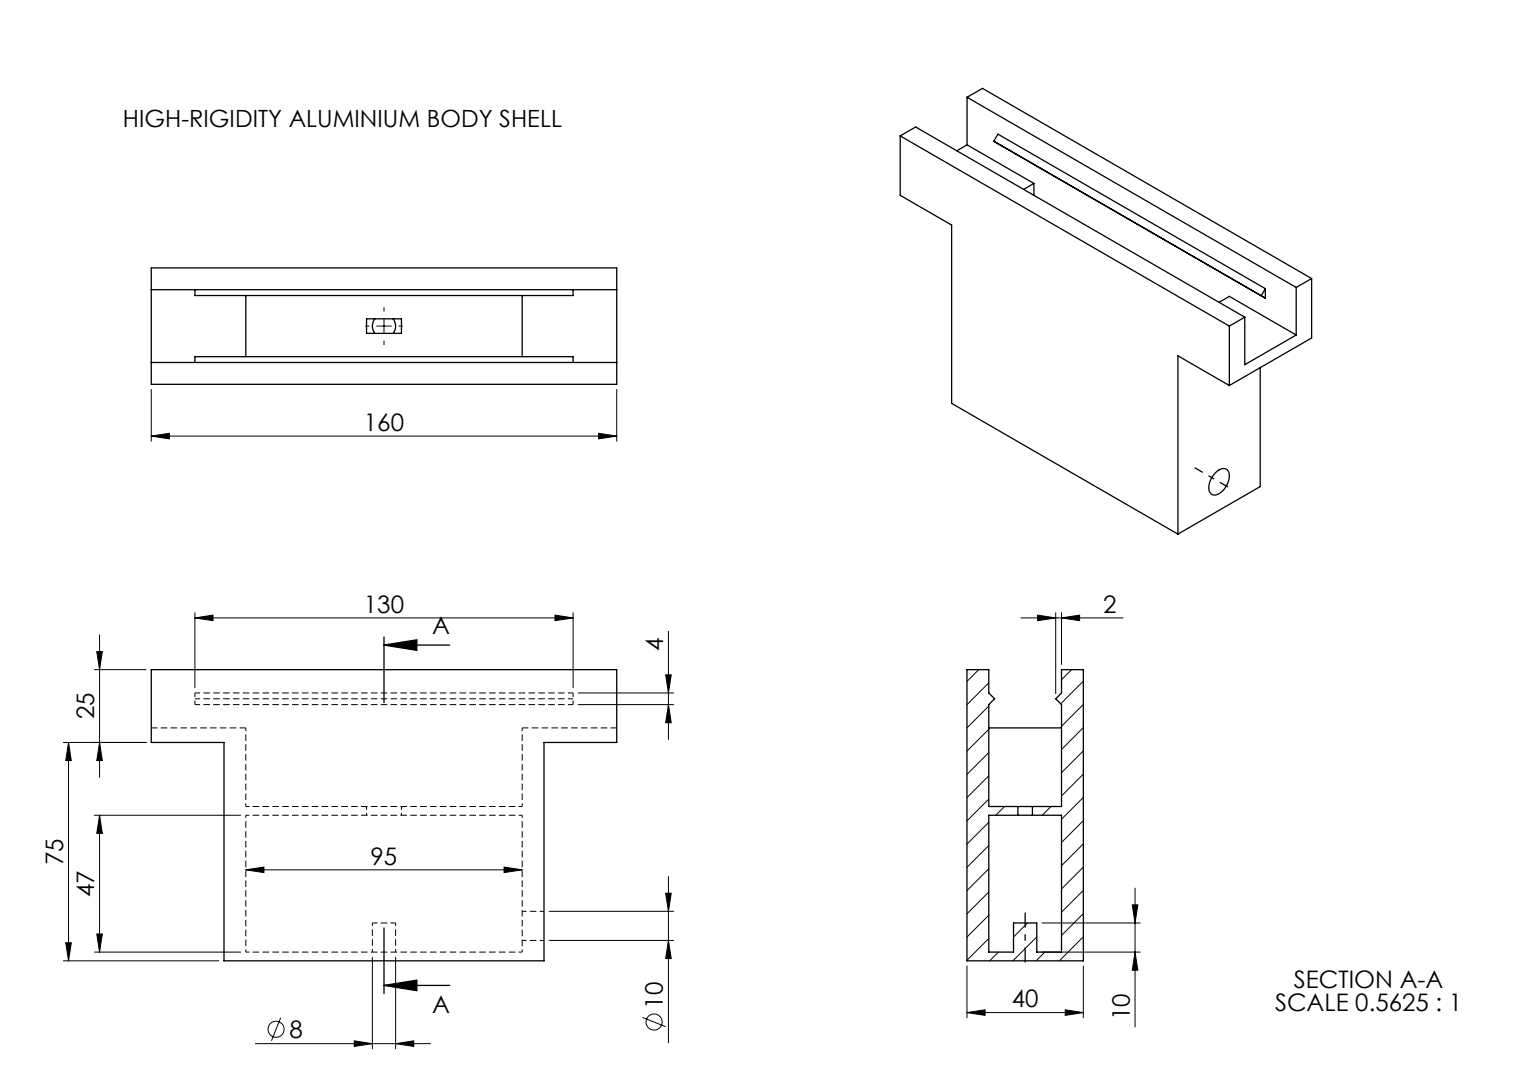
ISO-10303-21;
HEADER;
FILE_DESCRIPTION (('STEP AP214'),
    '1' );
FILE_NAME ('High-Rigidity Aluminium Body Shell.step',
    '2026-10-04T07:56:41',
    ( '' ),
    ( '' ),
    'SwSTEP 2.0',
    'SolidWorks 2026',
    '' );
FILE_SCHEMA (( 'AUTOMOTIVE_DESIGN' ));
ENDSEC;

DATA;
#5=LINE ( 'NONE', #7090, #369 ) ;
#14=LINE ( 'NONE', #7738, #5692 ) ;
#25=VECTOR ( 'NONE', #598, 1000.000000000000000 ) ;
#30=EDGE_LOOP ( 'NONE', ( #2065, #6214, #5997, #4915, #7865, #4258, #7605, #3266 ) ) ;
#39=CARTESIAN_POINT ( 'NONE',  ( -5.999999999999988454, -100.0010000000000048, -2.499999999999999112 ) ) ;
#47=FACE_OUTER_BOUND ( 'NONE', #854, .T. ) ;
#48=DIRECTION ( 'NONE',  ( -0.000000000000000000, 1.000000000000000000, 2.775557561562891351E-16 ) ) ;
#49=VECTOR ( 'NONE', #4022, 1000.000000000000000 ) ;
#50=AXIS2_PLACEMENT_3D ( 'NONE', #6623, #6543, #5905 ) ;
#52=EDGE_CURVE ( 'NONE', #1530, #5461, #2216, .T. ) ;
#56=ORIENTED_EDGE ( 'NONE', *, *, #5322, .F. ) ;
#58=LINE ( 'NONE', #6301, #4909 ) ;
#70=EDGE_CURVE ( 'NONE', #8240, #6658, #3048, .T. ) ;
#72=VERTEX_POINT ( 'NONE', #594 ) ;
#84=DIRECTION ( 'NONE',  ( 0.000000000000000000, -1.000000000000000000, -1.734723475976807094E-16 ) ) ;
#91=DIRECTION ( 'NONE',  ( 1.000000000000000000, -0.000000000000000000, -0.000000000000000000 ) ) ;
#94=ADVANCED_FACE ( 'NONE', ( #2381 ), #5021, .T. ) ;
#97=VERTEX_POINT ( 'NONE', #4421 ) ;
#98=AXIS2_PLACEMENT_3D ( 'NONE', #2797, #1653, #1018 ) ;
#107=LINE ( 'NONE', #2692, #5969 ) ;
#109=DIRECTION ( 'NONE',  ( -0.000000000000000000, 0.000000000000000000, -1.000000000000000000 ) ) ;
#113=EDGE_CURVE ( 'NONE', #4681, #4928, #8269, .T. ) ;
#114=ORIENTED_EDGE ( 'NONE', *, *, #1617, .T. ) ;
#119=ORIENTED_EDGE ( 'NONE', *, *, #70, .T. ) ;
#135=CARTESIAN_POINT ( 'NONE',  ( -65.00000000000000000, -7.999999999999992895, -12.50000000000000178 ) ) ;
#136=CARTESIAN_POINT ( 'NONE',  ( -65.00000000000000000, -12.00000000000000711, 12.49999999999999822 ) ) ;
#140=VERTEX_POINT ( 'NONE', #4384 ) ;
#145=CARTESIAN_POINT ( 'NONE',  ( -80.00000000000000000, -50.00000000000000711, -12.50000000000000888 ) ) ;
#146=CARTESIAN_POINT ( 'NONE',  ( 55.00000000000002132, -93.00000000000000000, 6.123233995736772199E-16 ) ) ;
#159=EDGE_LOOP ( 'NONE', ( #4079, #1702, #1986 ) ) ;
#160=FACE_OUTER_BOUND ( 'NONE', #6946, .T. ) ;
#167=EDGE_CURVE ( 'NONE', #2862, #1798, #3763, .T. ) ;
#170=CARTESIAN_POINT ( 'NONE',  ( 80.00000000000000000, 0.000000000000000000, 20.00000000000000000 ) ) ;
#176=CYLINDRICAL_SURFACE ( 'NONE', #6965, 5.000000000000004441 ) ;
#180=VECTOR ( 'NONE', #3060, 1000.000000000000000 ) ;
#184=VERTEX_POINT ( 'NONE', #4941 ) ;
#195=CARTESIAN_POINT ( 'NONE',  ( 80.00000000000000000, 0.000000000000000000, 20.00000000000000000 ) ) ;
#196=FILL_AREA_STYLE_COLOUR ( '', #1408 ) ;
#201=CARTESIAN_POINT ( 'NONE',  ( 80.00000000000000000, 0.000000000000000000, 20.00000000000000000 ) ) ;
#204=VERTEX_POINT ( 'NONE', #1706 ) ;
#211=DIRECTION ( 'NONE',  ( 9.251858538542971581E-17, -1.000000000000000000, 0.000000000000000000 ) ) ;
#216=CARTESIAN_POINT ( 'NONE',  ( -5.999999999999992895, -50.00000000000000000, -2.499999999999999112 ) ) ;
#217=DIRECTION ( 'NONE',  ( 0.000000000000000000, 0.7071067811865507924, -0.7071067811865441310 ) ) ;
#231=CARTESIAN_POINT ( 'NONE',  ( -80.00100000000001899, -83.00000000000002842, 0.000000000000000000 ) ) ;
#234=ORIENTED_EDGE ( 'NONE', *, *, #7378, .T. ) ;
#238=VERTEX_POINT ( 'NONE', #7087 ) ;
#239=DIRECTION ( 'NONE',  ( 0.000000000000000000, -0.000000000000000000, -1.000000000000000000 ) ) ;
#242=ORIENTED_EDGE ( 'NONE', *, *, #358, .F. ) ;
#251=FACE_OUTER_BOUND ( 'NONE', #7883, .T. ) ;
#255=AXIS2_PLACEMENT_3D ( 'NONE', #6696, #2244, #926 ) ;
#259=DIRECTION ( 'NONE',  ( 0.000000000000000000, 0.7071067811865442421, -0.7071067811865509034 ) ) ;
#262=ORIENTED_EDGE ( 'NONE', *, *, #5429, .F. ) ;
#267=VECTOR ( 'NONE', #2809, 1000.000000000000000 ) ;
#278=FILL_AREA_STYLE ('',( #196 ) ) ;
#281=ORIENTED_EDGE ( 'NONE', *, *, #3692, .F. ) ;
#282=DIRECTION ( 'NONE',  ( 0.000000000000000000, -2.775557561562891351E-16, 1.000000000000000000 ) ) ;
#285=ORIENTED_EDGE ( 'NONE', *, *, #8144, .T. ) ;
#303=FACE_OUTER_BOUND ( 'NONE', #1052, .T. ) ;
#308=ORIENTED_EDGE ( 'NONE', *, *, #7858, .F. ) ;
#312=CARTESIAN_POINT ( 'NONE',  ( -5.999999999999988454, -100.0010000000000048, 2.500000000000000888 ) ) ;
#320=ORIENTED_EDGE ( 'NONE', *, *, #4393, .F. ) ;
#321=CARTESIAN_POINT ( 'NONE',  ( 55.00000000000000000, -25.00000000000002132, 20.00000000000000000 ) ) ;
#339=CARTESIAN_POINT ( 'NONE',  ( 6.000000000000012434, -50.00000000000000000, 2.500000000000000888 ) ) ;
#343=ORIENTED_EDGE ( 'NONE', *, *, #113, .F. ) ;
#358=EDGE_CURVE ( 'NONE', #1800, #6097, #1314, .T. ) ;
#360=ORIENTED_EDGE ( 'NONE', *, *, #1284, .T. ) ;
#361=CYLINDRICAL_SURFACE ( 'NONE', #5299, 4.000000000000000000 ) ;
#369=VECTOR ( 'NONE', #5147, 1000.000000000000000 ) ;
#371=PRODUCT_CONTEXT ( 'NONE', #2292, 'mechanical' ) ;
#372=ORIENTED_EDGE ( 'NONE', *, *, #7078, .F. ) ;
#374=EDGE_CURVE ( 'NONE', #238, #5682, #7173, .T. ) ;
#375=ORIENTED_EDGE ( 'NONE', *, *, #3835, .T. ) ;
#379=LINE ( 'NONE', #7299, #1182 ) ;
#380=LINE ( 'NONE', #4853, #7186 ) ;
#382=CARTESIAN_POINT ( 'NONE',  ( -55.00000000000000000, -25.00000000000002132, 20.00000000000000000 ) ) ;
#383=EDGE_LOOP ( 'NONE', ( #4327, #3791, #8225, #2640 ) ) ;
#399=SURFACE_SIDE_STYLE ('',( #1115 ) ) ;
#401=ORIENTED_EDGE ( 'NONE', *, *, #6218, .F. ) ;
#403=ORIENTED_EDGE ( 'NONE', *, *, #1284, .F. ) ;
#415=ORIENTED_EDGE ( 'NONE', *, *, #5724, .T. ) ;
#416=CARTESIAN_POINT ( 'NONE',  ( 80.00000000000000000, 0.000000000000000000, 20.00000000000000000 ) ) ;
#421=DIRECTION ( 'NONE',  ( -1.261617073437677752E-16, 1.000000000000000000, 0.000000000000000000 ) ) ;
#434=DIRECTION ( 'NONE',  ( 0.000000000000000000, 0.000000000000000000, -1.000000000000000000 ) ) ;
#435=CIRCLE ( 'NONE', #50, 5.000000000000004441 ) ;
#438=EDGE_CURVE ( 'NONE', #4154, #6969, #4010, .T. ) ;
#442=EDGE_LOOP ( 'NONE', ( #7113, #2192, #7963, #2069 ) ) ;
#453=VECTOR ( 'NONE', #2497, 1000.000000000000000 ) ;
#455=EDGE_LOOP ( 'NONE', ( #5527, #7887, #7984, #6188 ) ) ;
#458=EDGE_LOOP ( 'NONE', ( #2051, #7413, #7304, #5700 ) ) ;
#467=ORIENTED_EDGE ( 'NONE', *, *, #5724, .F. ) ;
#483=LINE ( 'NONE', #2313, #180 ) ;
#493=ORIENTED_EDGE ( 'NONE', *, *, #657, .F. ) ;
#495=DIRECTION ( 'NONE',  ( -1.000000000000000000, -0.000000000000000000, -0.000000000000000000 ) ) ;
#508=EDGE_CURVE ( 'NONE', #4394, #4928, #3928, .T. ) ;
#525=DIRECTION ( 'NONE',  ( 1.261617073437677752E-16, -1.000000000000000000, -0.000000000000000000 ) ) ;
#550=DIRECTION ( 'NONE',  ( 0.000000000000000000, 0.000000000000000000, -1.000000000000000000 ) ) ;
#557=LINE ( 'NONE', #3220, #3294 ) ;
#578=LINE ( 'NONE', #2656, #3221 ) ;
#580=ORIENTED_EDGE ( 'NONE', *, *, #1489, .F. ) ;
#591=DIRECTION ( 'NONE',  ( -1.000000000000000000, -0.000000000000000000, -0.000000000000000000 ) ) ;
#594=CARTESIAN_POINT ( 'NONE',  ( -80.00000000000000000, 2.168404344971008868E-15, -12.50000000000000000 ) ) ;
#598=DIRECTION ( 'NONE',  ( -1.000000000000000000, -0.000000000000000000, -0.000000000000000000 ) ) ;
#604=VERTEX_POINT ( 'NONE', #826 ) ;
#613=CARTESIAN_POINT ( 'NONE',  ( -80.00000000000000000, -25.00000000000000000, 20.00000000000000000 ) ) ;
#619=CARTESIAN_POINT ( 'NONE',  ( -47.50000000000000711, -97.00000000000000000, 12.49999999999993960 ) ) ;
#628=CARTESIAN_POINT ( 'NONE',  ( 80.00000000000000000, 0.000000000000000000, 20.00000000000000000 ) ) ;
#636=LINE ( 'NONE', #5776, #2593 ) ;
#647=FACE_OUTER_BOUND ( 'NONE', #5300, .T. ) ;
#655=VECTOR ( 'NONE', #3803, 1000.000000000000000 ) ;
#657=EDGE_CURVE ( 'NONE', #72, #1757, #1333, .T. ) ;
#658=ORIENTED_EDGE ( 'NONE', *, *, #657, .T. ) ;
#659=FACE_BOUND ( 'NONE', #6052, .T. ) ;
#660=DIRECTION ( 'NONE',  ( -0.000000000000000000, -0.000000000000000000, -1.000000000000000000 ) ) ;
#669=EDGE_CURVE ( 'NONE', #1798, #1772, #3320, .T. ) ;
#681=CARTESIAN_POINT ( 'NONE',  ( -80.00000000000000000, 2.168404344971008868E-15, -12.50000000000000000 ) ) ;
#685=EDGE_LOOP ( 'NONE', ( #7292, #5717, #2988, #1427 ) ) ;
#687=CARTESIAN_POINT ( 'NONE',  ( 80.00000000000000000, -25.00000000000000000, 20.00000000000000000 ) ) ;
#688=CARTESIAN_POINT ( 'NONE',  ( -47.50000000000000711, -46.99999999999998579, -12.50000000000000888 ) ) ;
#702=CARTESIAN_POINT ( 'NONE',  ( -5.999999999999993783, -47.00000000000000000, -2.499999999999999112 ) ) ;
#716=VECTOR ( 'NONE', #6719, 1000.000000000000000 ) ;
#726=EDGE_CURVE ( 'NONE', #5175, #8255, #5334, .T. ) ;
#731=VERTEX_POINT ( 'NONE', #4655 ) ;
#747=LINE ( 'NONE', #4618, #7256 ) ;
#750=ORIENTED_EDGE ( 'NONE', *, *, #6561, .T. ) ;
#764=DIRECTION ( 'NONE',  ( -0.000000000000000000, -2.775557561562892337E-16, 1.000000000000000000 ) ) ;
#765=PLANE ( 'NONE',  #5548 ) ;
#769=ADVANCED_FACE ( 'NONE', ( #1502 ), #4069, .F. ) ;
#779=ADVANCED_FACE ( 'NONE', ( #5248 ), #6638, .F. ) ;
#792=CARTESIAN_POINT ( 'NONE',  ( 47.49999999999999289, -198.2344135219424857, 12.49999999999993960 ) ) ;
#794=ORIENTED_EDGE ( 'NONE', *, *, #5429, .T. ) ;
#806=EDGE_CURVE ( 'NONE', #6097, #3730, #5164, .T. ) ;
#807=LINE ( 'NONE', #39, #6725 ) ;
#821=DIRECTION ( 'NONE',  ( 1.000000000000000000, -0.000000000000000000, -0.000000000000000000 ) ) ;
#826=CARTESIAN_POINT ( 'NONE',  ( 80.00000000000000000, -25.00000000000000000, 20.00000000000000000 ) ) ;
#828=CARTESIAN_POINT ( 'NONE',  ( 80.00000000000000000, 2.168404344971008868E-15, -12.50000000000000000 ) ) ;
#843=EDGE_CURVE ( 'NONE', #7540, #3412, #107, .T. ) ;
#849=PLANE ( 'NONE',  #2666 ) ;
#850=CARTESIAN_POINT ( 'NONE',  ( 4.000000000000012434, -97.00000000000000000, 0.000000000000000000 ) ) ;
#854=EDGE_LOOP ( 'NONE', ( #4741, #415 ) ) ;
#861=CARTESIAN_POINT ( 'NONE',  ( 80.00000000000000000, 0.000000000000000000, 20.00000000000000000 ) ) ;
#864=VECTOR ( 'NONE', #7310, 1000.000000000000000 ) ;
#866=EDGE_CURVE ( 'NONE', #5004, #3412, #7048, .T. ) ;
#875=EDGE_LOOP ( 'NONE', ( #4314, #1494, #2609, #7246 ) ) ;
#888=FACE_OUTER_BOUND ( 'NONE', #2508, .T. ) ;
#894=LINE ( 'NONE', #136, #4759 ) ;
#898=ADVANCED_FACE ( 'NONE', ( #1362 ), #3345, .T. ) ;
#899=ORIENTED_EDGE ( 'NONE', *, *, #2957, .F. ) ;
#915=DIRECTION ( 'NONE',  ( 0.000000000000000000, 1.000000000000000000, 2.775557561562891351E-16 ) ) ;
#925=ORIENTED_EDGE ( 'NONE', *, *, #4635, .T. ) ;
#926=DIRECTION ( 'NONE',  ( -0.000000000000000000, 0.000000000000000000, -1.000000000000000000 ) ) ;
#932=VECTOR ( 'NONE', #2119, 1000.000000000000000 ) ;
#934=FACE_OUTER_BOUND ( 'NONE', #4950, .T. ) ;
#935=DIRECTION ( 'NONE',  ( 0.000000000000000000, -1.000000000000000000, 0.000000000000000000 ) ) ;
#948=DIRECTION ( 'NONE',  ( -1.000000000000000000, 0.000000000000000000, 0.000000000000000000 ) ) ;
#950=ADVANCED_FACE ( 'NONE', ( #47 ), #7770, .T. ) ;
#952=PLANE ( 'NONE',  #4975 ) ;
#954=ORIENTED_EDGE ( 'NONE', *, *, #8275, .F. ) ;
#956=ORIENTED_EDGE ( 'NONE', *, *, #4149, .T. ) ;
#961=ORIENTED_EDGE ( 'NONE', *, *, #806, .T. ) ;
#969=CARTESIAN_POINT ( 'NONE',  ( -5.999999999999988454, -100.0010000000000048, -2.499999999999999112 ) ) ;
#970=VERTEX_POINT ( 'NONE', #3218 ) ;
#974=EDGE_CURVE ( 'NONE', #4167, #3662, #5, .T. ) ;
#976=CARTESIAN_POINT ( 'NONE',  ( -80.00000000000000000, -47.00000000000000711, -12.50000000000000888 ) ) ;
#981=VERTEX_POINT ( 'NONE', #4551 ) ;
#982=LINE ( 'NONE', #2298, #7323 ) ;
#986=ORIENTED_EDGE ( 'NONE', *, *, #669, .T. ) ;
#991=EDGE_CURVE ( 'NONE', #2858, #7184, #5232, .T. ) ;
#994=VECTOR ( 'NONE', #495, 1000.000000000000000 ) ;
#1000=DIRECTION ( 'NONE',  ( -0.000000000000000000, 1.000000000000000000, 2.775557561562891351E-16 ) ) ;
#1012=VERTEX_POINT ( 'NONE', #135 ) ;
#1018=DIRECTION ( 'NONE',  ( 0.000000000000000000, -1.000000000000000000, -1.734723475976807094E-16 ) ) ;
#1023=EDGE_LOOP ( 'NONE', ( #7409, #4492, #6931, #3372 ) ) ;
#1024=CARTESIAN_POINT ( 'NONE',  ( 80.00000000000000000, 0.000000000000000000, -20.00000000000000000 ) ) ;
#1031=CARTESIAN_POINT ( 'NONE',  ( 47.49999999999999289, -46.99999999999998579, 12.49999999999998224 ) ) ;
#1032=ADVANCED_FACE ( 'NONE', ( #4469 ), #4594, .T. ) ;
#1034=( LENGTH_UNIT ( ) NAMED_UNIT ( * ) SI_UNIT ( .MILLI., .METRE. ) );
#1036=EDGE_LOOP ( 'NONE', ( #4830, #7266, #8107, #6146, #1939, #5954, #3636, #3435 ) ) ;
#1041=CARTESIAN_POINT ( 'NONE',  ( 1.223768561234547464E-14, -97.00000000000000000, 0.000000000000000000 ) ) ;
#1052=EDGE_LOOP ( 'NONE', ( #3029, #343, #320, #925 ) ) ;
#1062=EDGE_LOOP ( 'NONE', ( #5478, #3548, #403, #6706 ) ) ;
#1071=DIRECTION ( 'NONE',  ( -9.251858538542971581E-17, 1.000000000000000000, -0.000000000000000000 ) ) ;
#1076=ORIENTED_EDGE ( 'NONE', *, *, #1253, .F. ) ;
#1077=UNCERTAINTY_MEASURE_WITH_UNIT (LENGTH_MEASURE( 1.000000000000000082E-05 ), #5419, 'distance_accuracy_value', 'NONE');
#1090=ORIENTED_EDGE ( 'NONE', *, *, #3922, .T. ) ;
#1091=DIRECTION ( 'NONE',  ( -0.000000000000000000, -0.000000000000000000, -1.000000000000000000 ) ) ;
#1092=VERTEX_POINT ( 'NONE', #4012 ) ;
#1106=DIRECTION ( 'NONE',  ( -0.000000000000000000, -0.000000000000000000, -1.000000000000000000 ) ) ;
#1115=SURFACE_STYLE_FILL_AREA ( #8236 ) ;
#1118=ADVANCED_FACE ( 'NONE', ( #5950 ), #176, .F. ) ;
#1131=AXIS2_PLACEMENT_3D ( 'NONE', #7941, #259, #5193 ) ;
#1136=VERTEX_POINT ( 'NONE', #339 ) ;
#1158=PLANE ( 'NONE',  #2220 ) ;
#1162=VERTEX_POINT ( 'NONE', #216 ) ;
#1164=ADVANCED_FACE ( 'NONE', ( #4096, #7258 ), #4133, .F. ) ;
#1177=LINE ( 'NONE', #1816, #2009 ) ;
#1182=VECTOR ( 'NONE', #6075, 1000.000000000000000 ) ;
#1187=PLANE ( 'NONE',  #5298 ) ;
#1188=ORIENTED_EDGE ( 'NONE', *, *, #2399, .T. ) ;
#1189=LINE ( 'NONE', #3759, #453 ) ;
#1196=DIRECTION ( 'NONE',  ( 9.251858538542971581E-17, -1.000000000000000000, 0.000000000000000000 ) ) ;
#1197=VECTOR ( 'NONE', #5715, 1000.000000000000000 ) ;
#1202=VECTOR ( 'NONE', #84, 1000.000000000000000 ) ;
#1204=ADVANCED_FACE ( 'NONE', ( #1486 ), #849, .T. ) ;
#1206=VECTOR ( 'NONE', #2792, 1000.000000000000000 ) ;
#1232=DIRECTION ( 'NONE',  ( 0.000000000000000000, 0.000000000000000000, -1.000000000000000000 ) ) ;
#1245=CARTESIAN_POINT ( 'NONE',  ( -80.00000000000000000, -25.00000000000000000, 20.00000000000000000 ) ) ;
#1252=FACE_OUTER_BOUND ( 'NONE', #159, .T. ) ;
#1253=EDGE_CURVE ( 'NONE', #7447, #5257, #4677, .T. ) ;
#1260=ORIENTED_EDGE ( 'NONE', *, *, #358, .T. ) ;
#1275=DIRECTION ( 'NONE',  ( 0.000000000000000000, -1.000000000000000000, -1.734723475976807094E-16 ) ) ;
#1278=CARTESIAN_POINT ( 'NONE',  ( 55.00000000000000000, -25.00000000000002132, 20.00000000000000000 ) ) ;
#1279=CARTESIAN_POINT ( 'NONE',  ( -80.00000000000000000, -19.99999999999999645, -12.50000000000000355 ) ) ;
#1282=EDGE_LOOP ( 'NONE', ( #2510, #7406, #1561, #794 ) ) ;
#1284=EDGE_CURVE ( 'NONE', #6465, #5374, #5993, .T. ) ;
#1285=ORIENTED_EDGE ( 'NONE', *, *, #6456, .T. ) ;
#1300=LINE ( 'NONE', #619, #716 ) ;
#1314=LINE ( 'NONE', #3886, #1466 ) ;
#1318=LINE ( 'NONE', #3891, #25 ) ;
#1324=CARTESIAN_POINT ( 'NONE',  ( 80.00000000000000000, -25.00000000000000000, -20.00000000000000000 ) ) ;
#1331=VECTOR ( 'NONE', #6015, 1000.000000000000114 ) ;
#1333=LINE ( 'NONE', #4608, #1729 ) ;
#1336=LINE ( 'NONE', #1935, #7777 ) ;
#1341=VERTEX_POINT ( 'NONE', #6664 ) ;
#1342=LINE ( 'NONE', #702, #2282 ) ;
#1355=LINE ( 'NONE', #5898, #2705 ) ;
#1362=FACE_OUTER_BOUND ( 'NONE', #455, .T. ) ;
#1367=EDGE_LOOP ( 'NONE', ( #750, #4824, #5261, #5007 ) ) ;
#1370=CARTESIAN_POINT ( 'NONE',  ( -80.00000000000000000, 0.000000000000000000, 20.00000000000000000 ) ) ;
#1399=DIRECTION ( 'NONE',  ( -0.000000000000000000, -0.000000000000000000, -1.000000000000000000 ) ) ;
#1405=EDGE_CURVE ( 'NONE', #4928, #2966, #379, .T. ) ;
#1408=COLOUR_RGB ( '', 0.66274510, 0.83137255, 0.94901961) ;
#1412=DIRECTION ( 'NONE',  ( 1.000000000000000000, 9.251858538542971581E-17, 1.604941620322696727E-32 ) ) ;
#1422=CARTESIAN_POINT ( 'NONE',  ( -65.00000000000000000, -7.999999999999996447, 12.49999999999999822 ) ) ;
#1427=ORIENTED_EDGE ( 'NONE', *, *, #3922, .F. ) ;
#1431=ORIENTED_EDGE ( 'NONE', *, *, #1570, .T. ) ;
#1438=CARTESIAN_POINT ( 'NONE',  ( -80.00000000000000000, 2.168404344971008868E-15, -12.50000000000000000 ) ) ;
#1444=DIRECTION ( 'NONE',  ( 1.000000000000000000, 0.000000000000000000, 0.000000000000000000 ) ) ;
#1453=LINE ( 'NONE', #6594, #5169 ) ;
#1456=LINE ( 'NONE', #4028, #3228 ) ;
#1460=ADVANCED_FACE ( 'NONE', ( #934 ), #3467, .F. ) ;
#1466=VECTOR ( 'NONE', #1275, 1000.000000000000000 ) ;
#1467=ORIENTED_EDGE ( 'NONE', *, *, #3107, .T. ) ;
#1482=LINE ( 'NONE', #628, #7816 ) ;
#1486=FACE_OUTER_BOUND ( 'NONE', #1815, .T. ) ;
#1489=EDGE_CURVE ( 'NONE', #140, #2962, #8023, .T. ) ;
#1494=ORIENTED_EDGE ( 'NONE', *, *, #7223, .T. ) ;
#1502=FACE_OUTER_BOUND ( 'NONE', #6943, .T. ) ;
#1503=SURFACE_STYLE_FILL_AREA ( #278 ) ;
#1514=ADVANCED_FACE ( 'NONE', ( #4972 ), #1737, .F. ) ;
#1519=ORIENTED_EDGE ( 'NONE', *, *, #4696, .F. ) ;
#1521=DIRECTION ( 'NONE',  ( -1.000000000000000000, 0.000000000000000000, 0.000000000000000000 ) ) ;
#1522=FACE_OUTER_BOUND ( 'NONE', #685, .T. ) ;
#1529=AXIS2_PLACEMENT_3D ( 'NONE', #201, #8044, #239 ) ;
#1530=VERTEX_POINT ( 'NONE', #3713 ) ;
#1534=CIRCLE ( 'NONE', #5828, 4.000000000000000000 ) ;
#1550=ORIENTED_EDGE ( 'NONE', *, *, #4901, .F. ) ;
#1551=FACE_OUTER_BOUND ( 'NONE', #8281, .T. ) ;
#1554=VERTEX_POINT ( 'NONE', #6477 ) ;
#1561=ORIENTED_EDGE ( 'NONE', *, *, #167, .F. ) ;
#1570=EDGE_CURVE ( 'NONE', #1136, #981, #7746, .T. ) ;
#1571=UNCERTAINTY_MEASURE_WITH_UNIT (LENGTH_MEASURE( 1.000000000000000082E-05 ), #2347, 'distance_accuracy_value', 'NONE');
#1572=LINE ( 'NONE', #6791, #7584 ) ;
#1573=VERTEX_POINT ( 'NONE', #6434 ) ;
#1577=DIRECTION ( 'NONE',  ( -9.251858538542971581E-17, 1.000000000000000000, -0.000000000000000000 ) ) ;
#1582=EDGE_CURVE ( 'NONE', #7184, #3118, #1336, .T. ) ;
#1584=AXIS2_PLACEMENT_3D ( 'NONE', #3847, #5275, #1444 ) ;
#1588=( NAMED_UNIT ( * ) SI_UNIT ( $, .STERADIAN. ) SOLID_ANGLE_UNIT ( ) );
#1602=EDGE_LOOP ( 'NONE', ( #1188, #56, #2548, #7393 ) ) ;
#1609=ADVANCED_FACE ( 'NONE', ( #1252 ), #3947, .F. ) ;
#1610=VECTOR ( 'NONE', #6829, 1000.000000000000000 ) ;
#1617=EDGE_CURVE ( 'NONE', #3327, #7988, #5044, .T. ) ;
#1627=DIRECTION ( 'NONE',  ( -1.261617073437677752E-16, 1.000000000000000000, 0.000000000000000000 ) ) ;
#1633=DIRECTION ( 'NONE',  ( 0.000000000000000000, 0.7071067811865507924, -0.7071067811865441310 ) ) ;
#1635=DIRECTION ( 'NONE',  ( 0.000000000000000000, -1.000000000000000000, -1.734723475976807094E-16 ) ) ;
#1653=DIRECTION ( 'NONE',  ( 0.000000000000000000, -1.734723475976807094E-16, 1.000000000000000000 ) ) ;
#1663=VERTEX_POINT ( 'NONE', #3153 ) ;
#1668=ADVANCED_FACE ( 'NONE', ( #5709 ), #2518, .T. ) ;
#1679=DIRECTION ( 'NONE',  ( 1.000000000000000000, 0.000000000000000000, 0.000000000000000000 ) ) ;
#1687=ADVANCED_FACE ( 'NONE', ( #7025 ), #3824, .F. ) ;
#1692=FACE_OUTER_BOUND ( 'NONE', #30, .T. ) ;
#1702=ORIENTED_EDGE ( 'NONE', *, *, #2742, .F. ) ;
#1706=CARTESIAN_POINT ( 'NONE',  ( -65.00000000000000000, -12.00000000000000355, -12.50000000000000178 ) ) ;
#1729=VECTOR ( 'NONE', #7876, 1000.000000000000000 ) ;
#1737=PLANE ( 'NONE',  #3732 ) ;
#1742=FACE_OUTER_BOUND ( 'NONE', #1602, .T. ) ;
#1756=DIRECTION ( 'NONE',  ( 1.000000000000000000, 0.000000000000000000, 0.000000000000000000 ) ) ;
#1757=VERTEX_POINT ( 'NONE', #4071 ) ;
#1772=VERTEX_POINT ( 'NONE', #1422 ) ;
#1778=CARTESIAN_POINT ( 'NONE',  ( -54.99999999999999289, -100.0000000000000000, 20.00000000000000000 ) ) ;
#1783=CARTESIAN_POINT ( 'NONE',  ( 80.00000000000000000, -25.00000000000000000, 20.00000000000000000 ) ) ;
#1798=VERTEX_POINT ( 'NONE', #7959 ) ;
#1799=DIRECTION ( 'NONE',  ( -0.000000000000000000, 0.000000000000000000, 1.000000000000000000 ) ) ;
#1800=VERTEX_POINT ( 'NONE', #828 ) ;
#1802=DIRECTION ( 'NONE',  ( 1.000000000000000000, 1.261617073437677752E-16, 3.501690807976792361E-32 ) ) ;
#1815=EDGE_LOOP ( 'NONE', ( #2428, #308, #3461 ) ) ;
#1816=CARTESIAN_POINT ( 'NONE',  ( 65.00000000000000000, -9.999999999999994671, 10.50000000000000533 ) ) ;
#1826=CARTESIAN_POINT ( 'NONE',  ( -65.00000000000000000, -7.999999999999996447, 12.49999999999999822 ) ) ;
#1832=MANIFOLD_SOLID_BREP ( 'Cut-Extrude3', #1963 ) ;
#1844=ORIENTED_EDGE ( 'NONE', *, *, #4696, .T. ) ;
#1852=DIRECTION ( 'NONE',  ( -0.000000000000000000, 1.000000000000000000, 2.775557561562891351E-16 ) ) ;
#1863=AXIS2_PLACEMENT_3D ( 'NONE', #2604, #5880, #109 ) ;
#1878=VECTOR ( 'NONE', #1091, 1000.000000000000000 ) ;
#1880=EDGE_CURVE ( 'NONE', #5175, #2862, #2389, .T. ) ;
#1886=VECTOR ( 'NONE', #3859, 1000.000000000000000 ) ;
#1887=ORIENTED_EDGE ( 'NONE', *, *, #4926, .T. ) ;
#1888=CARTESIAN_POINT ( 'NONE',  ( 65.00000000000000000, -12.00000000000000355, -12.50000000000000178 ) ) ;
#1909=CARTESIAN_POINT ( 'NONE',  ( -80.00100000000001899, -93.00000000000004263, 6.123233995736772199E-16 ) ) ;
#1917=DIRECTION ( 'NONE',  ( 1.000000000000000000, 2.775557561562892337E-16, -0.000000000000000000 ) ) ;
#1935=CARTESIAN_POINT ( 'NONE',  ( 55.00000000000000000, -25.00000000000002132, 20.00000000000000000 ) ) ;
#1938=AXIS2_PLACEMENT_3D ( 'NONE', #2859, #915, #282 ) ;
#1939=ORIENTED_EDGE ( 'NONE', *, *, #7378, .F. ) ;
#1941=CARTESIAN_POINT ( 'NONE',  ( 65.00000000000000000, -7.999999999999992895, -12.50000000000000178 ) ) ;
#1962=DIRECTION ( 'NONE',  ( -1.000000000000000000, -1.261617073437677752E-16, -3.501690807976792361E-32 ) ) ;
#1963=CLOSED_SHELL ( 'NONE', ( #3411, #1032, #3271, #2345, #4211, #4487, #898, #6158, #3057, #5097, #7630, #779, #7010, #1164, #5712, #1460, #2041, #6132, #5943, #1687, #4380, #1514, #6128, #7098, #2710, #769, #5212, #5379, #94, #8306, #3727, #7921, #1668, #1609, #3609, #5284, #7576, #1204, #6288, #950, #1118 ) ) ;
#1968=CARTESIAN_POINT ( 'NONE',  ( 47.49999999999998579, -93.00000000000000000, 6.123233995736772199E-16 ) ) ;
#1970=DIRECTION ( 'NONE',  ( 0.000000000000000000, -0.000000000000000000, 1.000000000000000000 ) ) ;
#1983=DIRECTION ( 'NONE',  ( 0.000000000000000000, -1.000000000000000000, -1.734723475976807094E-16 ) ) ;
#1986=ORIENTED_EDGE ( 'NONE', *, *, #3601, .F. ) ;
#1995=CARTESIAN_POINT ( 'NONE',  ( 47.49999999999999289, -20.00000000000000355, 12.49999999999999112 ) ) ;
#2009=VECTOR ( 'NONE', #6944, 1000.000000000000000 ) ;
#2014=AXIS2_PLACEMENT_3D ( 'NONE', #8099, #2487, #4289 ) ;
#2041=ADVANCED_FACE ( 'NONE', ( #5501 ), #3649, .F. ) ;
#2051=ORIENTED_EDGE ( 'NONE', *, *, #6707, .F. ) ;
#2065=ORIENTED_EDGE ( 'NONE', *, *, #991, .T. ) ;
#2067=DIRECTION ( 'NONE',  ( -0.000000000000000000, 1.000000000000000000, 2.775557561562891351E-16 ) ) ;
#2069=ORIENTED_EDGE ( 'NONE', *, *, #2485, .T. ) ;
#2084=CARTESIAN_POINT ( 'NONE',  ( 55.00000000000002132, -82.99999999999998579, 0.000000000000000000 ) ) ;
#2095=CARTESIAN_POINT ( 'NONE',  ( 65.00000000000000000, -12.00000000000000355, -12.50000000000000178 ) ) ;
#2102=CARTESIAN_POINT ( 'NONE',  ( 65.00000000000000000, -7.999999999999996447, 12.49999999999999822 ) ) ;
#2119=DIRECTION ( 'NONE',  ( 1.000000000000000000, -0.000000000000000000, -0.000000000000000000 ) ) ;
#2124=DIRECTION ( 'NONE',  ( 1.000000000000000000, 9.251858538542971581E-17, 1.604941620322696727E-32 ) ) ;
#2133=ORIENTED_EDGE ( 'NONE', *, *, #5412, .F. ) ;
#2134=VECTOR ( 'NONE', #1852, 1000.000000000000000 ) ;
#2136=DIRECTION ( 'NONE',  ( -1.000000000000000000, -0.000000000000000000, -0.000000000000000000 ) ) ;
#2153=VERTEX_POINT ( 'NONE', #1968 ) ;
#2160=EDGE_LOOP ( 'NONE', ( #467, #6260, #1887, #3569 ) ) ;
#2162=PLANE ( 'NONE',  #7408 ) ;
#2171=EDGE_CURVE ( 'NONE', #5374, #2526, #3101, .T. ) ;
#2175=EDGE_LOOP ( 'NONE', ( #5491, #5086, #7142, #7162 ) ) ;
#2177=LINE ( 'NONE', #5411, #864 ) ;
#2192=ORIENTED_EDGE ( 'NONE', *, *, #70, .F. ) ;
#2201=LINE ( 'NONE', #3538, #932 ) ;
#2208=LINE ( 'NONE', #2839, #2619 ) ;
#2212=AXIS2_PLACEMENT_3D ( 'NONE', #321, #3995, #6684 ) ;
#2216=LINE ( 'NONE', #7351, #7943 ) ;
#2218=VECTOR ( 'NONE', #1071, 1000.000000000000000 ) ;
#2220=AXIS2_PLACEMENT_3D ( 'NONE', #6296, #1196, #7091 ) ;
#2222=AXIS2_PLACEMENT_3D ( 'NONE', #3044, #591, #550 ) ;
#2225=DIRECTION ( 'NONE',  ( -0.000000000000000000, -0.7071067811865507924, -0.7071067811865441310 ) ) ;
#2242=EDGE_CURVE ( 'NONE', #7184, #604, #2591, .T. ) ;
#2244=DIRECTION ( 'NONE',  ( 1.000000000000000000, 0.000000000000000000, -0.000000000000000000 ) ) ;
#2250=CARTESIAN_POINT ( 'NONE',  ( -80.00000000000000000, -47.00000000000000711, 12.49999999999999289 ) ) ;
#2256=DIRECTION ( 'NONE',  ( 1.000000000000000000, 0.000000000000000000, 0.000000000000000000 ) ) ;
#2263=DIRECTION ( 'NONE',  ( 0.000000000000000000, 0.000000000000000000, -1.000000000000000000 ) ) ;
#2266=CARTESIAN_POINT ( 'NONE',  ( 47.49999999999999289, -198.2344135219424857, -12.50000000000005151 ) ) ;
#2281=EDGE_CURVE ( 'NONE', #2962, #7308, #3774, .T. ) ;
#2282=VECTOR ( 'NONE', #6481, 1000.000000000000000 ) ;
#2283=ORIENTED_EDGE ( 'NONE', *, *, #7691, .T. ) ;
#2291=DIRECTION ( 'NONE',  ( 0.000000000000000000, 0.000000000000000000, 1.000000000000000000 ) ) ;
#2292=APPLICATION_CONTEXT ( 'automotive_design' ) ;
#2296=DIRECTION ( 'NONE',  ( 0.000000000000000000, 0.000000000000000000, -1.000000000000000000 ) ) ;
#2298=CARTESIAN_POINT ( 'NONE',  ( -80.00000000000000000, -2.168404344971008868E-15, 12.50000000000000000 ) ) ;
#2306=CARTESIAN_POINT ( 'NONE',  ( 6.000000000000007105, -50.00000000000000000, -2.499999999999999112 ) ) ;
#2311=DIRECTION ( 'NONE',  ( -1.000000000000000000, 0.000000000000000000, -0.000000000000000000 ) ) ;
#2313=CARTESIAN_POINT ( 'NONE',  ( -80.00000000000000000, -25.00000000000000000, -20.00000000000000000 ) ) ;
#2324=CARTESIAN_POINT ( 'NONE',  ( 6.000000000000006217, -47.00000000000000000, -2.499999999999999112 ) ) ;
#2343=AXIS2_PLACEMENT_3D ( 'NONE', #3856, #7147, #7610 ) ;
#2345=ADVANCED_FACE ( 'NONE', ( #5658, #7099 ), #6345, .T. ) ;
#2347=( LENGTH_UNIT ( ) NAMED_UNIT ( * ) SI_UNIT ( .MILLI., .METRE. ) );
#2352=UNCERTAINTY_MEASURE_WITH_UNIT (LENGTH_MEASURE( 1.000000000000000082E-05 ), #1034, 'distance_accuracy_value', 'NONE');
#2355=ORIENTED_EDGE ( 'NONE', *, *, #3890, .T. ) ;
#2367=ORIENTED_EDGE ( 'NONE', *, *, #3717, .T. ) ;
#2375=FACE_OUTER_BOUND ( 'NONE', #3074, .T. ) ;
#2376=ORIENTED_EDGE ( 'NONE', *, *, #7403, .F. ) ;
#2381=FACE_OUTER_BOUND ( 'NONE', #1036, .T. ) ;
#2389=LINE ( 'NONE', #4991, #7200 ) ;
#2391=DIRECTION ( 'NONE',  ( -1.261617073437677752E-16, 1.000000000000000000, 0.000000000000000000 ) ) ;
#2399=EDGE_CURVE ( 'NONE', #3118, #4154, #5737, .T. ) ;
#2404=CARTESIAN_POINT ( 'NONE',  ( 80.00000000000000000, -25.00000000000000000, 20.00000000000000000 ) ) ;
#2413=ORIENTED_EDGE ( 'NONE', *, *, #6523, .F. ) ;
#2419=CARTESIAN_POINT ( 'NONE',  ( -80.00000000000000000, -50.00000000000000711, 12.49999999999999289 ) ) ;
#2423=PLANE ( 'NONE',  #5437 ) ;
#2426=VECTOR ( 'NONE', #7312, 1000.000000000000000 ) ;
#2428=ORIENTED_EDGE ( 'NONE', *, *, #3717, .F. ) ;
#2429=EDGE_CURVE ( 'NONE', #1573, #7540, #58, .T. ) ;
#2432=FACE_OUTER_BOUND ( 'NONE', #3201, .T. ) ;
#2442=ORIENTED_EDGE ( 'NONE', *, *, #4590, .T. ) ;
#2443=FACE_OUTER_BOUND ( 'NONE', #1282, .T. ) ;
#2458=EDGE_CURVE ( 'NONE', #7988, #8240, #7187, .T. ) ;
#2464=DIRECTION ( 'NONE',  ( 0.000000000000000000, 0.000000000000000000, -1.000000000000000000 ) ) ;
#2485=EDGE_CURVE ( 'NONE', #7988, #2655, #5329, .T. ) ;
#2487=DIRECTION ( 'NONE',  ( 0.000000000000000000, 0.000000000000000000, -1.000000000000000000 ) ) ;
#2496=EDGE_LOOP ( 'NONE', ( #6830, #3490, #8007, #2721 ) ) ;
#2497=DIRECTION ( 'NONE',  ( -0.000000000000000000, 1.000000000000000000, 2.775557561562891351E-16 ) ) ;
#2508=EDGE_LOOP ( 'NONE', ( #7523, #6131, #8016, #5417 ) ) ;
#2510=ORIENTED_EDGE ( 'NONE', *, *, #4629, .T. ) ;
#2518=PLANE ( 'NONE',  #5073 ) ;
#2526=VERTEX_POINT ( 'NONE', #3477 ) ;
#2543=DIRECTION ( 'NONE',  ( 0.000000000000000000, -2.775557561562891351E-16, 1.000000000000000000 ) ) ;
#2548=ORIENTED_EDGE ( 'NONE', *, *, #2242, .F. ) ;
#2553=VECTOR ( 'NONE', #4545, 1000.000000000000000 ) ;
#2567=EDGE_LOOP ( 'NONE', ( #1431, #3511, #2951, #899 ) ) ;
#2568=CARTESIAN_POINT ( 'NONE',  ( -3.999999999999988898, -87.00000000000001421, 4.898587196589412829E-16 ) ) ;
#2570=ORIENTED_EDGE ( 'NONE', *, *, #6134, .T. ) ;
#2577=DIRECTION ( 'NONE',  ( 1.000000000000000000, -0.000000000000000000, -0.000000000000000000 ) ) ;
#2591=LINE ( 'NONE', #687, #3960 ) ;
#2593=VECTOR ( 'NONE', #1962, 1000.000000000000000 ) ;
#2601=DIRECTION ( 'NONE',  ( -9.251858538542971581E-17, 1.000000000000000000, 0.000000000000000000 ) ) ;
#2603=APPLICATION_CONTEXT ( 'automotive_design' ) ;
#2604=CARTESIAN_POINT ( 'NONE',  ( -65.00000000000000000, 0.000000000000000000, 0.000000000000000000 ) ) ;
#2608=VECTOR ( 'NONE', #3187, 1000.000000000000000 ) ;
#2609=ORIENTED_EDGE ( 'NONE', *, *, #843, .T. ) ;
#2619=VECTOR ( 'NONE', #935, 1000.000000000000000 ) ;
#2626=EDGE_CURVE ( 'NONE', #1554, #204, #7868, .T. ) ;
#2627=CARTESIAN_POINT ( 'NONE',  ( 65.00000000000000000, 0.000000000000000000, 0.000000000000000000 ) ) ;
#2640=ORIENTED_EDGE ( 'NONE', *, *, #113, .T. ) ;
#2643=LINE ( 'NONE', #1888, #6776 ) ;
#2654=EDGE_CURVE ( 'NONE', #5682, #970, #1453, .T. ) ;
#2655=VERTEX_POINT ( 'NONE', #3401 ) ;
#2656=CARTESIAN_POINT ( 'NONE',  ( -5.999999999999992895, -50.00000000000000000, -2.499999999999999112 ) ) ;
#2665=LINE ( 'NONE', #1438, #3761 ) ;
#2666=AXIS2_PLACEMENT_3D ( 'NONE', #3430, #2838, #6745 ) ;
#2680=EDGE_LOOP ( 'NONE', ( #281, #7421 ) ) ;
#2683=CIRCLE ( 'NONE', #5901, 4.000000000000000000 ) ;
#2692=CARTESIAN_POINT ( 'NONE',  ( -47.50000000000000711, -20.00000000000000355, 12.49999999999999112 ) ) ;
#2705=VECTOR ( 'NONE', #7719, 1000.000000000000000 ) ;
#2710=ADVANCED_FACE ( 'NONE', ( #5869 ), #6507, .F. ) ;
#2711=CARTESIAN_POINT ( 'NONE',  ( -54.99999999999999289, -100.0000000000000000, 20.00000000000000000 ) ) ;
#2712=CARTESIAN_POINT ( 'NONE',  ( -5.999999999999993783, -47.00000000000000000, -2.499999999999999112 ) ) ;
#2717=CARTESIAN_POINT ( 'NONE',  ( 1.097606853890779561E-14, -87.00000000000001421, 0.000000000000000000 ) ) ;
#2721=ORIENTED_EDGE ( 'NONE', *, *, #3407, .T. ) ;
#2742=EDGE_CURVE ( 'NONE', #1012, #2766, #2177, .T. ) ;
#2748=VECTOR ( 'NONE', #1802, 1000.000000000000000 ) ;
#2750=CARTESIAN_POINT ( 'NONE',  ( 1.223768561234547464E-14, -97.00000000000000000, 0.000000000000000000 ) ) ;
#2753=VECTOR ( 'NONE', #2296, 1000.000000000000000 ) ;
#2766=VERTEX_POINT ( 'NONE', #6800 ) ;
#2775=SURFACE_STYLE_USAGE ( .BOTH. , #6641 ) ;
#2790=ORIENTED_EDGE ( 'NONE', *, *, #7003, .F. ) ;
#2792=DIRECTION ( 'NONE',  ( -0.000000000000000000, -0.000000000000000000, -1.000000000000000000 ) ) ;
#2795=EDGE_CURVE ( 'NONE', #4167, #731, #1534, .T. ) ;
#2797=CARTESIAN_POINT ( 'NONE',  ( -80.00000000000000000, -2.168404344971008868E-15, 12.50000000000000000 ) ) ;
#2799=LINE ( 'NONE', #3431, #7705 ) ;
#2809=DIRECTION ( 'NONE',  ( -0.000000000000000000, 1.000000000000000000, 2.775557561562891351E-16 ) ) ;
#2821=EDGE_CURVE ( 'NONE', #1663, #5257, #8117, .T. ) ;
#2832=DIRECTION ( 'NONE',  ( 0.000000000000000000, 0.000000000000000000, 1.000000000000000000 ) ) ;
#2834=CARTESIAN_POINT ( 'NONE',  ( -80.00000000000000000, -25.00000000000000000, 20.00000000000000000 ) ) ;
#2838=DIRECTION ( 'NONE',  ( -1.000000000000000000, 0.000000000000000000, -0.000000000000000000 ) ) ;
#2839=CARTESIAN_POINT ( 'NONE',  ( -80.00000000000000000, 0.000000000000000000, -20.00000000000000000 ) ) ;
#2840=AXIS2_PLACEMENT_3D ( 'NONE', #8120, #5497, #1756 ) ;
#2858=VERTEX_POINT ( 'NONE', #8036 ) ;
#2859=CARTESIAN_POINT ( 'NONE',  ( -80.00000000000000000, -19.99999999999999645, -12.50000000000000355 ) ) ;
#2862=VERTEX_POINT ( 'NONE', #6880 ) ;
#2891=CARTESIAN_POINT ( 'NONE',  ( 1.097606853890779561E-14, -87.00000000000001421, 0.000000000000000000 ) ) ;
#2892=MECHANICAL_DESIGN_GEOMETRIC_PRESENTATION_REPRESENTATION('',(#8272),#3693);
#2900=CARTESIAN_POINT ( 'NONE',  ( -65.00000000000000000, -12.00000000000000355, -12.50000000000000178 ) ) ;
#2930=CARTESIAN_POINT ( 'NONE',  ( 55.00000000000002132, -99.99999999999998579, -20.00000000000000000 ) ) ;
#2932=VECTOR ( 'NONE', #2291, 1000.000000000000000 ) ;
#2938=PLANE ( 'NONE',  #6906 ) ;
#2948=SHAPE_DEFINITION_REPRESENTATION ( #3596, #7093 ) ;
#2951=ORIENTED_EDGE ( 'NONE', *, *, #52, .F. ) ;
#2954=VECTOR ( 'NONE', #6953, 1000.000000000000000 ) ;
#2957=EDGE_CURVE ( 'NONE', #1136, #1530, #4147, .T. ) ;
#2962=VERTEX_POINT ( 'NONE', #1031 ) ;
#2966=VERTEX_POINT ( 'NONE', #2930 ) ;
#2977=EDGE_LOOP ( 'NONE', ( #4835, #6883, #3718, #3019 ) ) ;
#2988=ORIENTED_EDGE ( 'NONE', *, *, #1570, .F. ) ;
#2989=LINE ( 'NONE', #3031, #7659 ) ;
#2990=ORIENTED_EDGE ( 'NONE', *, *, #7078, .T. ) ;
#3000=CARTESIAN_POINT ( 'NONE',  ( 55.00000000000000000, -25.00000000000002132, 20.00000000000000000 ) ) ;
#3008=DIRECTION ( 'NONE',  ( -1.000000000000000000, 0.000000000000000000, -0.000000000000000000 ) ) ;
#3014=ORIENTED_EDGE ( 'NONE', *, *, #6561, .F. ) ;
#3019=ORIENTED_EDGE ( 'NONE', *, *, #7634, .T. ) ;
#3029=ORIENTED_EDGE ( 'NONE', *, *, #508, .T. ) ;
#3031=CARTESIAN_POINT ( 'NONE',  ( -80.00000000000000000, -19.99999999999999645, -12.50000000000000355 ) ) ;
#3044=CARTESIAN_POINT ( 'NONE',  ( 47.49999999999998579, -88.00000000000000000, 0.000000000000000000 ) ) ;
#3048=LINE ( 'NONE', #2419, #655 ) ;
#3057=ADVANCED_FACE ( 'NONE', ( #7482 ), #2423, .F. ) ;
#3058=VECTOR ( 'NONE', #4488, 1000.000000000000000 ) ;
#3060=DIRECTION ( 'NONE',  ( 1.000000000000000000, -8.326672684688674053E-16, 0.000000000000000000 ) ) ;
#3074=EDGE_LOOP ( 'NONE', ( #114, #4062, #4119, #3349 ) ) ;
#3079=AXIS2_PLACEMENT_3D ( 'NONE', #969, #8017, #211 ) ;
#3086=VECTOR ( 'NONE', #7916, 1000.000000000000000 ) ;
#3101=LINE ( 'NONE', #6467, #7463 ) ;
#3107=EDGE_CURVE ( 'NONE', #72, #1573, #3767, .T. ) ;
#3118=VERTEX_POINT ( 'NONE', #4388 ) ;
#3125=LINE ( 'NONE', #5057, #1610 ) ;
#3127=DIRECTION ( 'NONE',  ( -1.000000000000000000, -8.326672684688674053E-16, 0.000000000000000000 ) ) ;
#3135=FACE_BOUND ( 'NONE', #4685, .T. ) ;
#3153=CARTESIAN_POINT ( 'NONE',  ( -5.999999999999992895, -50.00000000000000000, 2.500000000000001776 ) ) ;
#3158=ORIENTED_EDGE ( 'NONE', *, *, #3359, .T. ) ;
#3187=DIRECTION ( 'NONE',  ( 1.000000000000000000, 1.261617073437677752E-16, 0.000000000000000000 ) ) ;
#3194=DIRECTION ( 'NONE',  ( 8.326672684688674053E-16, 1.000000000000000000, -0.000000000000000000 ) ) ;
#3195=CARTESIAN_POINT ( 'NONE',  ( 6.000000000000011546, -100.0010000000000048, 2.500000000000000888 ) ) ;
#3201=EDGE_LOOP ( 'NONE', ( #3500, #119, #5362, #3158 ) ) ;
#3204=AXIS2_PLACEMENT_3D ( 'NONE', #681, #5775, #7814 ) ;
#3211=DIRECTION ( 'NONE',  ( -0.000000000000000000, 1.000000000000000000, -0.000000000000000000 ) ) ;
#3218=CARTESIAN_POINT ( 'NONE',  ( 80.00000000000000000, -2.168404344971008868E-15, 12.50000000000000000 ) ) ;
#3219=EDGE_CURVE ( 'NONE', #1573, #5004, #6417, .T. ) ;
#3220=CARTESIAN_POINT ( 'NONE',  ( 47.49999999999999289, -198.2344135219424857, 12.49999999999993960 ) ) ;
#3221=VECTOR ( 'NONE', #7751, 1000.000000000000000 ) ;
#3228=VECTOR ( 'NONE', #2225, 1000.000000000000114 ) ;
#3234=DIRECTION ( 'NONE',  ( -1.000000000000000000, -0.000000000000000000, -0.000000000000000000 ) ) ;
#3241=ORIENTED_EDGE ( 'NONE', *, *, #6456, .F. ) ;
#3242=FACE_OUTER_BOUND ( 'NONE', #3565, .T. ) ;
#3266=ORIENTED_EDGE ( 'NONE', *, *, #6508, .T. ) ;
#3269=EDGE_CURVE ( 'NONE', #2962, #5374, #6925, .T. ) ;
#3271=ADVANCED_FACE ( 'NONE', ( #3726, #3135 ), #1158, .T. ) ;
#3272=LINE ( 'NONE', #1370, #7722 ) ;
#3284=VECTOR ( 'NONE', #4315, 1000.000000000000000 ) ;
#3285=EDGE_LOOP ( 'NONE', ( #580, #956, #8162, #2790, #4169, #3956, #6303, #6820 ) ) ;
#3286=DIRECTION ( 'NONE',  ( 1.000000000000000000, -8.326672684688674053E-16, 0.000000000000000000 ) ) ;
#3294=VECTOR ( 'NONE', #48, 1000.000000000000000 ) ;
#3306=DIRECTION ( 'NONE',  ( -2.775557561562892337E-16, 1.000000000000000000, -0.000000000000000000 ) ) ;
#3307=CARTESIAN_POINT ( 'NONE',  ( 55.00000000000002132, -88.00000000000000000, 0.000000000000000000 ) ) ;
#3313=CARTESIAN_POINT ( 'NONE',  ( -47.50000000000000711, -49.99999999999998579, 12.49999999999993960 ) ) ;
#3315=LINE ( 'NONE', #5830, #2608 ) ;
#3317=DIRECTION ( 'NONE',  ( 0.000000000000000000, -0.7071067811865466846, -0.7071067811865484609 ) ) ;
#3320=LINE ( 'NONE', #2102, #6828 ) ;
#3325=EDGE_CURVE ( 'NONE', #4798, #6658, #557, .T. ) ;
#3327=VERTEX_POINT ( 'NONE', #3848 ) ;
#3345=PLANE ( 'NONE',  #3204 ) ;
#3349=ORIENTED_EDGE ( 'NONE', *, *, #4025, .T. ) ;
#3359=EDGE_CURVE ( 'NONE', #4798, #5382, #636, .T. ) ;
#3372=ORIENTED_EDGE ( 'NONE', *, *, #5640, .F. ) ;
#3376=ORIENTED_EDGE ( 'NONE', *, *, #1880, .T. ) ;
#3387=DIRECTION ( 'NONE',  ( -9.251858538542971581E-17, 1.000000000000000000, -0.000000000000000000 ) ) ;
#3401=CARTESIAN_POINT ( 'NONE',  ( 47.50000000000000000, -49.99999999999999289, -12.50000000000000888 ) ) ;
#3407=EDGE_CURVE ( 'NONE', #97, #2766, #1318, .T. ) ;
#3411=ADVANCED_FACE ( 'NONE', ( #8314 ), #5276, .F. ) ;
#3412=VERTEX_POINT ( 'NONE', #3468 ) ;
#3426=AXIS2_PLACEMENT_3D ( 'NONE', #382, #3510, #8027 ) ;
#3428=CIRCLE ( 'NONE', #2222, 5.000000000000004441 ) ;
#3430=CARTESIAN_POINT ( 'NONE',  ( -65.00000000000000000, 0.000000000000000000, 0.000000000000000000 ) ) ;
#3431=CARTESIAN_POINT ( 'NONE',  ( -65.00000000000000000, -12.00000000000000355, -12.50000000000000178 ) ) ;
#3435=ORIENTED_EDGE ( 'NONE', *, *, #3835, .F. ) ;
#3441=DIRECTION ( 'NONE',  ( -1.000000000000000000, 0.000000000000000000, 0.000000000000000000 ) ) ;
#3446=EDGE_LOOP ( 'NONE', ( #5213, #6347, #7281, #2570 ) ) ;
#3451=FACE_OUTER_BOUND ( 'NONE', #6987, .T. ) ;
#3461=ORIENTED_EDGE ( 'NONE', *, *, #4629, .F. ) ;
#3463=LINE ( 'NONE', #5520, #5915 ) ;
#3467=PLANE ( 'NONE',  #7371 ) ;
#3468=CARTESIAN_POINT ( 'NONE',  ( -47.50000000000000711, -20.00000000000000355, 12.49999999999999112 ) ) ;
#3472=EDGE_CURVE ( 'NONE', #6782, #3690, #6891, .T. ) ;
#3475=ORIENTED_EDGE ( 'NONE', *, *, #1880, .F. ) ;
#3477=CARTESIAN_POINT ( 'NONE',  ( 47.49999999999999289, -19.99999999999999645, -12.50000000000000000 ) ) ;
#3485=ORIENTED_EDGE ( 'NONE', *, *, #5515, .F. ) ;
#3490=ORIENTED_EDGE ( 'NONE', *, *, #2626, .F. ) ;
#3500=ORIENTED_EDGE ( 'NONE', *, *, #6196, .T. ) ;
#3505=DIRECTION ( 'NONE',  ( 1.000000000000000000, 0.000000000000000000, 0.000000000000000000 ) ) ;
#3506=PRODUCT_DEFINITION ( 'UNKNOWN', '', #7807, #6790 ) ;
#3510=DIRECTION ( 'NONE',  ( 1.000000000000000000, 9.251858538542972814E-17, -0.000000000000000000 ) ) ;
#3511=ORIENTED_EDGE ( 'NONE', *, *, #5697, .T. ) ;
#3538=CARTESIAN_POINT ( 'NONE',  ( -80.00000000000000000, -20.00000000000000355, 12.49999999999999645 ) ) ;
#3539=ORIENTED_EDGE ( 'NONE', *, *, #1582, .F. ) ;
#3548=ORIENTED_EDGE ( 'NONE', *, *, #3269, .T. ) ;
#3549=FACE_BOUND ( 'NONE', #4600, .T. ) ;
#3553=EDGE_LOOP ( 'NONE', ( #961, #8296, #2133, #4075, #4703, #7206, #401, #1260 ) ) ;
#3561=FILL_AREA_STYLE_COLOUR ( '', #8083 ) ;
#3565=EDGE_LOOP ( 'NONE', ( #5016, #360, #3777, #7028, #242, #1519, #1467, #7503 ) ) ;
#3566=FACE_OUTER_BOUND ( 'NONE', #3446, .T. ) ;
#3569=ORIENTED_EDGE ( 'NONE', *, *, #974, .F. ) ;
#3579=ORIENTED_EDGE ( 'NONE', *, *, #3325, .T. ) ;
#3587=CARTESIAN_POINT ( 'NONE',  ( 80.00000000000000000, -20.00000000000000355, 12.49999999999999645 ) ) ;
#3596=PRODUCT_DEFINITION_SHAPE ( 'NONE', 'NONE',  #3506 ) ;
#3601=EDGE_CURVE ( 'NONE', #204, #1012, #2799, .T. ) ;
#3603=VECTOR ( 'NONE', #2124, 1000.000000000000000 ) ;
#3604=( NAMED_UNIT ( * ) PLANE_ANGLE_UNIT ( ) SI_UNIT ( $, .RADIAN. ) );
#3606=ORIENTED_EDGE ( 'NONE', *, *, #167, .T. ) ;
#3609=ADVANCED_FACE ( 'NONE', ( #7857 ), #765, .F. ) ;
#3636=ORIENTED_EDGE ( 'NONE', *, *, #2399, .F. ) ;
#3648=ORIENTED_EDGE ( 'NONE', *, *, #2171, .F. ) ;
#3649=PLANE ( 'NONE',  #5699 ) ;
#3651=CARTESIAN_POINT ( 'NONE',  ( -47.50000000000000711, -198.2344135219424857, 12.49999999999993960 ) ) ;
#3662=VERTEX_POINT ( 'NONE', #850 ) ;
#3684=VECTOR ( 'NONE', #2067, 1000.000000000000000 ) ;
#3690=VERTEX_POINT ( 'NONE', #2084 ) ;
#3692=EDGE_CURVE ( 'NONE', #3690, #6782, #435, .T. ) ;
#3693=( GEOMETRIC_REPRESENTATION_CONTEXT ( 3 ) GLOBAL_UNCERTAINTY_ASSIGNED_CONTEXT ( ( #1077 ) ) GLOBAL_UNIT_ASSIGNED_CONTEXT ( ( #5419, #4610, #1588 ) ) REPRESENTATION_CONTEXT ( 'NONE', 'WORKASPACE' ) );
#3706=CARTESIAN_POINT ( 'NONE',  ( -5.999999999999993783, -47.00000000000000000, 2.500000000000000888 ) ) ;
#3708=ORIENTED_EDGE ( 'NONE', *, *, #5412, .T. ) ;
#3713=CARTESIAN_POINT ( 'NONE',  ( 6.000000000000012434, -50.00000000000000000, -2.499999999999999112 ) ) ;
#3717=EDGE_CURVE ( 'NONE', #8255, #184, #894, .T. ) ;
#3718=ORIENTED_EDGE ( 'NONE', *, *, #5762, .F. ) ;
#3726=FACE_OUTER_BOUND ( 'NONE', #442, .T. ) ;
#3727=ADVANCED_FACE ( 'NONE', ( #6034 ), #4639, .F. ) ;
#3730=VERTEX_POINT ( 'NONE', #3587 ) ;
#3732=AXIS2_PLACEMENT_3D ( 'NONE', #1778, #421, #7507 ) ;
#3751=VECTOR ( 'NONE', #7106, 1000.000000000000000 ) ;
#3753=VECTOR ( 'NONE', #2832, 1000.000000000000000 ) ;
#3759=CARTESIAN_POINT ( 'NONE',  ( -47.50000000000000711, -198.2344135219424857, -12.50000000000005151 ) ) ;
#3761=VECTOR ( 'NONE', #2577, 1000.000000000000000 ) ;
#3763=LINE ( 'NONE', #5569, #4827 ) ;
#3767=LINE ( 'NONE', #6964, #8264 ) ;
#3774=LINE ( 'NONE', #5033, #6781 ) ;
#3777=ORIENTED_EDGE ( 'NONE', *, *, #2171, .T. ) ;
#3791=ORIENTED_EDGE ( 'NONE', *, *, #3890, .F. ) ;
#3794=EDGE_CURVE ( 'NONE', #1757, #1341, #2208, .T. ) ;
#3799=CARTESIAN_POINT ( 'NONE',  ( -5.999999999999992895, -50.00000000000000000, -2.499999999999999112 ) ) ;
#3800=PLANE ( 'NONE',  #5832 ) ;
#3803=DIRECTION ( 'NONE',  ( 1.000000000000000000, 9.251858538542971581E-17, 1.604941620322696727E-32 ) ) ;
#3811=DIRECTION ( 'NONE',  ( 1.000000000000000000, 8.326672684688674053E-16, -0.000000000000000000 ) ) ;
#3824=PLANE ( 'NONE',  #4672 ) ;
#3829=ORIENTED_EDGE ( 'NONE', *, *, #4472, .T. ) ;
#3830=DIRECTION ( 'NONE',  ( 0.000000000000000000, -1.734723475976807094E-16, 1.000000000000000000 ) ) ;
#3831=CARTESIAN_POINT ( 'NONE',  ( 55.00000000000002132, -99.99999999999998579, 20.00000000000000000 ) ) ;
#3835=EDGE_CURVE ( 'NONE', #2966, #3118, #380, .T. ) ;
#3844=CARTESIAN_POINT ( 'NONE',  ( 80.00000000000000000, 0.000000000000000000, -20.00000000000000000 ) ) ;
#3847=CARTESIAN_POINT ( 'NONE',  ( 1.097606853890779561E-14, -87.00000000000001421, 0.000000000000000000 ) ) ;
#3848=CARTESIAN_POINT ( 'NONE',  ( -47.50000000000000711, -97.00000000000000000, -12.50000000000002309 ) ) ;
#3851=ORIENTED_EDGE ( 'NONE', *, *, #4049, .T. ) ;
#3856=CARTESIAN_POINT ( 'NONE',  ( 47.49999999999998579, -88.00000000000000000, 0.000000000000000000 ) ) ;
#3859=DIRECTION ( 'NONE',  ( -0.000000000000000000, -1.000000000000000000, -0.000000000000000000 ) ) ;
#3869=LINE ( 'NONE', #5845, #1197 ) ;
#3882=PLANE ( 'NONE',  #4036 ) ;
#3886=CARTESIAN_POINT ( 'NONE',  ( 80.00000000000000000, 2.168404344971008868E-15, -12.50000000000000000 ) ) ;
#3890=EDGE_CURVE ( 'NONE', #2858, #2966, #5049, .T. ) ;
#3891=CARTESIAN_POINT ( 'NONE',  ( 65.00000000000000000, -9.999999999999991118, -10.50000000000000888 ) ) ;
#3909=( GEOMETRIC_REPRESENTATION_CONTEXT ( 3 ) GLOBAL_UNCERTAINTY_ASSIGNED_CONTEXT ( ( #1571 ) ) GLOBAL_UNIT_ASSIGNED_CONTEXT ( ( #2347, #3604, #4913 ) ) REPRESENTATION_CONTEXT ( 'NONE', 'WORKASPACE' ) );
#3922=EDGE_CURVE ( 'NONE', #1663, #1136, #4450, .T. ) ;
#3928=LINE ( 'NONE', #5103, #4650 ) ;
#3947=PLANE ( 'NONE',  #1863 ) ;
#3954=FACE_OUTER_BOUND ( 'NONE', #6546, .T. ) ;
#3956=ORIENTED_EDGE ( 'NONE', *, *, #4829, .T. ) ;
#3960=VECTOR ( 'NONE', #7779, 1000.000000000000000 ) ;
#3985=CARTESIAN_POINT ( 'NONE',  ( 47.49999999999999289, -96.99999999999998579, -12.50000000000002309 ) ) ;
#3995=DIRECTION ( 'NONE',  ( -1.000000000000000000, -2.775557561562892337E-16, 0.000000000000000000 ) ) ;
#4010=LINE ( 'NONE', #3844, #8289 ) ;
#4012=CARTESIAN_POINT ( 'NONE',  ( 47.49999999999998579, -82.99999999999998579, 0.000000000000000000 ) ) ;
#4013=DIRECTION ( 'NONE',  ( -0.000000000000000000, 0.7071067811865442421, 0.7071067811865509034 ) ) ;
#4022=DIRECTION ( 'NONE',  ( 0.000000000000000000, 0.000000000000000000, 1.000000000000000000 ) ) ;
#4025=EDGE_CURVE ( 'NONE', #5382, #3327, #1300, .T. ) ;
#4028=CARTESIAN_POINT ( 'NONE',  ( 65.00000000000000000, -12.00000000000000355, -12.50000000000000178 ) ) ;
#4030=VECTOR ( 'NONE', #6370, 1000.000000000000000 ) ;
#4036=AXIS2_PLACEMENT_3D ( 'NONE', #2627, #4129, #4848 ) ;
#4049=EDGE_CURVE ( 'NONE', #4845, #1012, #4494, .T. ) ;
#4054=DIRECTION ( 'NONE',  ( 0.000000000000000000, 1.000000000000000000, 0.000000000000000000 ) ) ;
#4062=ORIENTED_EDGE ( 'NONE', *, *, #2458, .T. ) ;
#4069=PLANE ( 'NONE',  #5235 ) ;
#4071=CARTESIAN_POINT ( 'NONE',  ( -80.00000000000000000, 0.000000000000000000, -20.00000000000000000 ) ) ;
#4075=ORIENTED_EDGE ( 'NONE', *, *, #7555, .F. ) ;
#4076=CARTESIAN_POINT ( 'NONE',  ( 80.00000000000000000, -19.99999999999999645, -12.50000000000000355 ) ) ;
#4079=ORIENTED_EDGE ( 'NONE', *, *, #5897, .F. ) ;
#4096=FACE_BOUND ( 'NONE', #4448, .T. ) ;
#4100=DIRECTION ( 'NONE',  ( 9.251858538542972814E-17, -1.000000000000000000, 0.000000000000000000 ) ) ;
#4109=DIRECTION ( 'NONE',  ( 0.000000000000000000, 1.000000000000000000, 2.775557561562891351E-16 ) ) ;
#4115=PLANE ( 'NONE',  #2212 ) ;
#4119=ORIENTED_EDGE ( 'NONE', *, *, #6196, .F. ) ;
#4126=ORIENTED_EDGE ( 'NONE', *, *, #4926, .F. ) ;
#4128=PRODUCT ( 'High-Rigidity Aluminium Body Shell', 'High-Rigidity Aluminium Body Shell', '', ( #371 ) ) ;
#4129=DIRECTION ( 'NONE',  ( -1.000000000000000000, 0.000000000000000000, -0.000000000000000000 ) ) ;
#4133=PLANE ( 'NONE',  #98 ) ;
#4147=LINE ( 'NONE', #2306, #6510 ) ;
#4149=EDGE_CURVE ( 'NONE', #140, #3412, #4576, .T. ) ;
#4150=CARTESIAN_POINT ( 'NONE',  ( -65.00000000000000000, -12.00000000000000711, 12.49999999999999822 ) ) ;
#4154=VERTEX_POINT ( 'NONE', #5215 ) ;
#4167=VERTEX_POINT ( 'NONE', #7795 ) ;
#4169=ORIENTED_EDGE ( 'NONE', *, *, #2654, .T. ) ;
#4194=ORIENTED_EDGE ( 'NONE', *, *, #7858, .T. ) ;
#4206=EDGE_LOOP ( 'NONE', ( #3014, #372 ) ) ;
#4211=ADVANCED_FACE ( 'NONE', ( #7244, #3954 ), #6016, .F. ) ;
#4217=CARTESIAN_POINT ( 'NONE',  ( 47.49999999999999289, -49.99999999999998579, 12.49999999999993960 ) ) ;
#4219=ORIENTED_EDGE ( 'NONE', *, *, #2281, .T. ) ;
#4239=CARTESIAN_POINT ( 'NONE',  ( -80.00000000000000000, -2.168404344971008868E-15, 12.50000000000000000 ) ) ;
#4258=ORIENTED_EDGE ( 'NONE', *, *, #5762, .T. ) ;
#4259=LINE ( 'NONE', #8029, #7458 ) ;
#4287=AXIS2_PLACEMENT_3D ( 'NONE', #8294, #3830, #1983 ) ;
#4289=DIRECTION ( 'NONE',  ( -1.000000000000000000, 0.000000000000000000, -0.000000000000000000 ) ) ;
#4311=( NAMED_UNIT ( * ) SI_UNIT ( $, .STERADIAN. ) SOLID_ANGLE_UNIT ( ) );
#4314=ORIENTED_EDGE ( 'NONE', *, *, #4992, .F. ) ;
#4315=DIRECTION ( 'NONE',  ( -0.000000000000000000, -0.000000000000000000, -1.000000000000000000 ) ) ;
#4327=ORIENTED_EDGE ( 'NONE', *, *, #1405, .T. ) ;
#4337=DIRECTION ( 'NONE',  ( -0.000000000000000000, 0.000000000000000000, 1.000000000000000000 ) ) ;
#4343=DIRECTION ( 'NONE',  ( -1.000000000000000000, 0.000000000000000000, -0.000000000000000000 ) ) ;
#4354=AXIS2_PLACEMENT_3D ( 'NONE', #8108, #4902, #7474 ) ;
#4368=ORIENTED_EDGE ( 'NONE', *, *, #7634, .F. ) ;
#4369=CARTESIAN_POINT ( 'NONE',  ( 65.00000000000000000, -7.999999999999996447, 12.49999999999999822 ) ) ;
#4380=ADVANCED_FACE ( 'NONE', ( #303 ), #4513, .F. ) ;
#4384=CARTESIAN_POINT ( 'NONE',  ( -47.50000000000000711, -46.99999999999998579, 12.49999999999999112 ) ) ;
#4388=CARTESIAN_POINT ( 'NONE',  ( 55.00000000000000000, -25.00000000000002132, -20.00000000000000000 ) ) ;
#4393=EDGE_CURVE ( 'NONE', #7734, #4681, #1572, .T. ) ;
#4394=VERTEX_POINT ( 'NONE', #5361 ) ;
#4406=DIRECTION ( 'NONE',  ( -0.000000000000000000, -0.000000000000000000, -1.000000000000000000 ) ) ;
#4413=AXIS2_PLACEMENT_3D ( 'NONE', #4369, #7541, #8214 ) ;
#4421=CARTESIAN_POINT ( 'NONE',  ( 65.00000000000000000, -9.999999999999991118, -10.50000000000000888 ) ) ;
#4448=EDGE_LOOP ( 'NONE', ( #6609, #986, #4194, #6804 ) ) ;
#4449=CARTESIAN_POINT ( 'NONE',  ( -80.00000000000000000, -2.168404344971008868E-15, 12.50000000000000000 ) ) ;
#4450=LINE ( 'NONE', #6439, #8259 ) ;
#4469=FACE_OUTER_BOUND ( 'NONE', #2160, .T. ) ;
#4472=EDGE_CURVE ( 'NONE', #6658, #2655, #5486, .T. ) ;
#4487=ADVANCED_FACE ( 'NONE', ( #2375 ), #1187, .F. ) ;
#4488=DIRECTION ( 'NONE',  ( -9.251858538542971581E-17, 1.000000000000000000, -0.000000000000000000 ) ) ;
#4492=ORIENTED_EDGE ( 'NONE', *, *, #5753, .T. ) ;
#4494=LINE ( 'NONE', #1941, #994 ) ;
#4513=PLANE ( 'NONE',  #3426 ) ;
#4532=ORIENTED_EDGE ( 'NONE', *, *, #2742, .T. ) ;
#4533=CARTESIAN_POINT ( 'NONE',  ( 1.097606853890779561E-14, -87.00000000000001421, 0.000000000000000000 ) ) ;
#4545=DIRECTION ( 'NONE',  ( -1.000000000000000000, 0.000000000000000000, 0.000000000000000000 ) ) ;
#4551=CARTESIAN_POINT ( 'NONE',  ( 6.000000000000006217, -47.00000000000000000, 2.500000000000000888 ) ) ;
#4552=DIRECTION ( 'NONE',  ( 0.000000000000000000, 1.000000000000000000, 0.000000000000000000 ) ) ;
#4560=DIRECTION ( 'NONE',  ( -0.000000000000000000, 1.000000000000000000, 2.775557561562891351E-16 ) ) ;
#4562=DIRECTION ( 'NONE',  ( 0.000000000000000000, 1.000000000000000000, 0.000000000000000000 ) ) ;
#4576=LINE ( 'NONE', #6566, #3684 ) ;
#4590=EDGE_CURVE ( 'NONE', #1162, #1663, #5681, .T. ) ;
#4594=CYLINDRICAL_SURFACE ( 'NONE', #1584, 4.000000000000000000 ) ;
#4600=EDGE_LOOP ( 'NONE', ( #6668, #8043, #1076, #5565 ) ) ;
#4608=CARTESIAN_POINT ( 'NONE',  ( -80.00000000000000000, 0.000000000000000000, 20.00000000000000000 ) ) ;
#4610=( NAMED_UNIT ( * ) PLANE_ANGLE_UNIT ( ) SI_UNIT ( $, .RADIAN. ) );
#4618=CARTESIAN_POINT ( 'NONE',  ( -80.00000000000000000, -25.00000000000000000, 20.00000000000000000 ) ) ;
#4629=EDGE_CURVE ( 'NONE', #184, #1772, #8265, .T. ) ;
#4635=EDGE_CURVE ( 'NONE', #7734, #4394, #3125, .T. ) ;
#4639=PLANE ( 'NONE',  #1131 ) ;
#4650=VECTOR ( 'NONE', #6496, 1000.000000000000000 ) ;
#4655=CARTESIAN_POINT ( 'NONE',  ( -3.999999999999988898, -87.00000000000001421, 4.898587196589413815E-16 ) ) ;
#4672=AXIS2_PLACEMENT_3D ( 'NONE', #613, #3194, #6558 ) ;
#4677=LINE ( 'NONE', #7381, #2932 ) ;
#4681=VERTEX_POINT ( 'NONE', #2711 ) ;
#4685=EDGE_LOOP ( 'NONE', ( #1090, #6014, #8148, #2442 ) ) ;
#4689=VECTOR ( 'NONE', #1106, 1000.000000000000000 ) ;
#4692=CARTESIAN_POINT ( 'NONE',  ( -80.00000000000000000, -19.99999999999999645, -12.50000000000000355 ) ) ;
#4696=EDGE_CURVE ( 'NONE', #72, #1800, #2665, .T. ) ;
#4703=ORIENTED_EDGE ( 'NONE', *, *, #5322, .T. ) ;
#4704=PLANE ( 'NONE',  #1529 ) ;
#4705=DIRECTION ( 'NONE',  ( 1.000000000000000000, 0.000000000000000000, 0.000000000000000000 ) ) ;
#4715=DIRECTION ( 'NONE',  ( -0.000000000000000000, 0.000000000000000000, 1.000000000000000000 ) ) ;
#4722=EDGE_CURVE ( 'NONE', #5453, #238, #6410, .T. ) ;
#4733=CARTESIAN_POINT ( 'NONE',  ( -47.50000000000000711, -49.99999999999998579, 12.49999999999998224 ) ) ;
#4741=ORIENTED_EDGE ( 'NONE', *, *, #2795, .T. ) ;
#4759=VECTOR ( 'NONE', #217, 1000.000000000000114 ) ;
#4798=VERTEX_POINT ( 'NONE', #7083 ) ;
#4799=CARTESIAN_POINT ( 'NONE',  ( -54.99999999999999289, -100.0000000000000000, -20.00000000000000000 ) ) ;
#4805=DIRECTION ( 'NONE',  ( 1.000000000000000000, 9.251858538542971581E-17, 1.604941620322696727E-32 ) ) ;
#4815=ORIENTED_EDGE ( 'NONE', *, *, #6218, .T. ) ;
#4824=ORIENTED_EDGE ( 'NONE', *, *, #4901, .T. ) ;
#4827=VECTOR ( 'NONE', #4906, 1000.000000000000000 ) ;
#4829=EDGE_CURVE ( 'NONE', #970, #3730, #5896, .T. ) ;
#4830=ORIENTED_EDGE ( 'NONE', *, *, #1405, .F. ) ;
#4835=ORIENTED_EDGE ( 'NONE', *, *, #6258, .T. ) ;
#4845=VERTEX_POINT ( 'NONE', #7763 ) ;
#4846=PLANE ( 'NONE',  #255 ) ;
#4847=MECHANICAL_DESIGN_GEOMETRIC_PRESENTATION_REPRESENTATION('',(#6998),#3909);
#4848=DIRECTION ( 'NONE',  ( -0.000000000000000000, 0.000000000000000000, 1.000000000000000000 ) ) ;
#4853=CARTESIAN_POINT ( 'NONE',  ( 55.00000000000000000, -25.00000000000002132, -20.00000000000000000 ) ) ;
#4859=PLANE ( 'NONE',  #4354 ) ;
#4877=DIRECTION ( 'NONE',  ( -1.000000000000000000, 0.000000000000000000, 0.000000000000000000 ) ) ;
#4889=ORIENTED_EDGE ( 'NONE', *, *, #4722, .F. ) ;
#4890=LINE ( 'NONE', #2834, #1206 ) ;
#4901=EDGE_CURVE ( 'NONE', #2153, #6782, #7677, .T. ) ;
#4902=DIRECTION ( 'NONE',  ( 9.251858538542971581E-17, -1.000000000000000000, 0.000000000000000000 ) ) ;
#4906=DIRECTION ( 'NONE',  ( -0.000000000000000000, 0.7071067811865484609, 0.7071067811865465735 ) ) ;
#4909=VECTOR ( 'NONE', #5698, 1000.000000000000000 ) ;
#4913=( NAMED_UNIT ( * ) SI_UNIT ( $, .STERADIAN. ) SOLID_ANGLE_UNIT ( ) );
#4915=ORIENTED_EDGE ( 'NONE', *, *, #4722, .T. ) ;
#4926=EDGE_CURVE ( 'NONE', #7486, #3662, #6046, .T. ) ;
#4928=VERTEX_POINT ( 'NONE', #4799 ) ;
#4930=ORIENTED_EDGE ( 'NONE', *, *, #991, .F. ) ;
#4941=CARTESIAN_POINT ( 'NONE',  ( -65.00000000000000000, -9.999999999999994671, 10.50000000000000533 ) ) ;
#4950=EDGE_LOOP ( 'NONE', ( #7754, #4219, #7967, #3648 ) ) ;
#4972=FACE_OUTER_BOUND ( 'NONE', #383, .T. ) ;
#4975=AXIS2_PLACEMENT_3D ( 'NONE', #4692, #4109, #7954 ) ;
#4982=( GEOMETRIC_REPRESENTATION_CONTEXT ( 3 ) GLOBAL_UNCERTAINTY_ASSIGNED_CONTEXT ( ( #2352 ) ) GLOBAL_UNIT_ASSIGNED_CONTEXT ( ( #1034, #5538, #4311 ) ) REPRESENTATION_CONTEXT ( 'NONE', 'WORKASPACE' ) );
#4991=CARTESIAN_POINT ( 'NONE',  ( 65.00000000000000000, -12.00000000000000711, 12.49999999999999822 ) ) ;
#4992=EDGE_CURVE ( 'NONE', #6465, #140, #7422, .T. ) ;
#5004=VERTEX_POINT ( 'NONE', #7374 ) ;
#5007=ORIENTED_EDGE ( 'NONE', *, *, #8335, .F. ) ;
#5016=ORIENTED_EDGE ( 'NONE', *, *, #7223, .F. ) ;
#5021=PLANE ( 'NONE',  #7396 ) ;
#5031=VECTOR ( 'NONE', #3811, 1000.000000000000000 ) ;
#5033=CARTESIAN_POINT ( 'NONE',  ( 47.49999999999999289, -198.2344135219424857, 12.49999999999993960 ) ) ;
#5044=LINE ( 'NONE', #5749, #2134 ) ;
#5049=LINE ( 'NONE', #3831, #6775 ) ;
#5057=CARTESIAN_POINT ( 'NONE',  ( -55.00000000000000000, -25.00000000000002132, 20.00000000000000000 ) ) ;
#5058=ORIENTED_EDGE ( 'NONE', *, *, #806, .F. ) ;
#5071=DIRECTION ( 'NONE',  ( -1.000000000000000000, -1.261617073437677752E-16, 0.000000000000000000 ) ) ;
#5073=AXIS2_PLACEMENT_3D ( 'NONE', #5082, #5793, #7662 ) ;
#5075=DIRECTION ( 'NONE',  ( 0.000000000000000000, -1.000000000000000000, 0.000000000000000000 ) ) ;
#5082=CARTESIAN_POINT ( 'NONE',  ( 65.00000000000000000, 0.000000000000000000, 0.000000000000000000 ) ) ;
#5086=ORIENTED_EDGE ( 'NONE', *, *, #2429, .F. ) ;
#5089=ORIENTED_EDGE ( 'NONE', *, *, #5458, .F. ) ;
#5094=VECTOR ( 'NONE', #7623, 1000.000000000000000 ) ;
#5097=ADVANCED_FACE ( 'NONE', ( #888 ), #5311, .F. ) ;
#5103=CARTESIAN_POINT ( 'NONE',  ( -55.00000000000000000, -25.00000000000002132, -20.00000000000000000 ) ) ;
#5116=ORIENTED_EDGE ( 'NONE', *, *, #726, .T. ) ;
#5147=DIRECTION ( 'NONE',  ( 1.261617073437677752E-16, -1.000000000000000000, -0.000000000000000000 ) ) ;
#5154=DIRECTION ( 'NONE',  ( -1.261617073437677752E-16, 1.000000000000000000, 0.000000000000000000 ) ) ;
#5156=AXIS2_PLACEMENT_3D ( 'NONE', #861, #3441, #6674 ) ;
#5164=LINE ( 'NONE', #7743, #3751 ) ;
#5169=VECTOR ( 'NONE', #821, 1000.000000000000000 ) ;
#5171=ORIENTED_EDGE ( 'NONE', *, *, #3794, .T. ) ;
#5175=VERTEX_POINT ( 'NONE', #7293 ) ;
#5184=EDGE_CURVE ( 'NONE', #7308, #3730, #2201, .T. ) ;
#5189=DIRECTION ( 'NONE',  ( -0.000000000000000000, 1.000000000000000000, -0.000000000000000000 ) ) ;
#5192=DIRECTION ( 'NONE',  ( -1.261617073437677752E-16, 1.000000000000000000, 0.000000000000000000 ) ) ;
#5193=DIRECTION ( 'NONE',  ( 0.000000000000000000, 0.7071067811865507924, 0.7071067811865441310 ) ) ;
#5202=DIRECTION ( 'NONE',  ( 0.000000000000000000, 0.7071067811865483499, -0.7071067811865465735 ) ) ;
#5205=CARTESIAN_POINT ( 'NONE',  ( 65.00000000000000000, -12.00000000000000711, 12.49999999999999822 ) ) ;
#5212=ADVANCED_FACE ( 'NONE', ( #251 ), #4846, .F. ) ;
#5213=ORIENTED_EDGE ( 'NONE', *, *, #5522, .F. ) ;
#5215=CARTESIAN_POINT ( 'NONE',  ( 80.00000000000000000, -25.00000000000000000, -20.00000000000000000 ) ) ;
#5232=LINE ( 'NONE', #1278, #6297 ) ;
#5233=DIRECTION ( 'NONE',  ( 0.000000000000000000, 1.000000000000000000, 0.000000000000000000 ) ) ;
#5235=AXIS2_PLACEMENT_3D ( 'NONE', #195, #7152, #6556 ) ;
#5245=CARTESIAN_POINT ( 'NONE',  ( -47.50000000000000711, -49.99999999999998579, -12.50000000000001954 ) ) ;
#5248=FACE_OUTER_BOUND ( 'NONE', #2567, .T. ) ;
#5257=VERTEX_POINT ( 'NONE', #3706 ) ;
#5261=ORIENTED_EDGE ( 'NONE', *, *, #3472, .T. ) ;
#5275=DIRECTION ( 'NONE',  ( 1.261617073437677752E-16, -1.000000000000000000, -0.000000000000000000 ) ) ;
#5276=CYLINDRICAL_SURFACE ( 'NONE', #6626, 5.000000000000004441 ) ;
#5284=ADVANCED_FACE ( 'NONE', ( #2443 ), #6232, .F. ) ;
#5298=AXIS2_PLACEMENT_3D ( 'NONE', #7550, #6243, #4337 ) ;
#5299=AXIS2_PLACEMENT_3D ( 'NONE', #6886, #525, #1679 ) ;
#5300=EDGE_LOOP ( 'NONE', ( #4532, #5349, #2376, #3851 ) ) ;
#5311=PLANE ( 'NONE',  #3079 ) ;
#5318=CARTESIAN_POINT ( 'NONE',  ( -80.00100000000001899, -88.00000000000004263, 0.000000000000000000 ) ) ;
#5322=EDGE_CURVE ( 'NONE', #604, #4154, #6276, .T. ) ;
#5327=ORIENTED_EDGE ( 'NONE', *, *, #6707, .T. ) ;
#5329=LINE ( 'NONE', #145, #7054 ) ;
#5334=LINE ( 'NONE', #5205, #3086 ) ;
#5349=ORIENTED_EDGE ( 'NONE', *, *, #3407, .F. ) ;
#5358=DIRECTION ( 'NONE',  ( 0.000000000000000000, -0.7071067811865507924, 0.7071067811865441310 ) ) ;
#5361=CARTESIAN_POINT ( 'NONE',  ( -55.00000000000000000, -25.00000000000002132, -20.00000000000000000 ) ) ;
#5362=ORIENTED_EDGE ( 'NONE', *, *, #3325, .F. ) ;
#5374=VERTEX_POINT ( 'NONE', #7462 ) ;
#5379=ADVANCED_FACE ( 'NONE', ( #1692 ), #6819, .F. ) ;
#5382=VERTEX_POINT ( 'NONE', #7578 ) ;
#5393=ORIENTED_EDGE ( 'NONE', *, *, #5184, .T. ) ;
#5399=CARTESIAN_POINT ( 'NONE',  ( 47.49999999999999289, -198.2344135219424857, 12.49999999999993960 ) ) ;
#5411=CARTESIAN_POINT ( 'NONE',  ( -65.00000000000000000, -7.999999999999992895, -12.50000000000000178 ) ) ;
#5412=EDGE_CURVE ( 'NONE', #5453, #970, #5593, .T. ) ;
#5414=LINE ( 'NONE', #231, #2426 ) ;
#5417=ORIENTED_EDGE ( 'NONE', *, *, #4590, .F. ) ;
#5418=AXIS2_PLACEMENT_3D ( 'NONE', #3307, #7221, #4552 ) ;
#5419=( LENGTH_UNIT ( ) NAMED_UNIT ( * ) SI_UNIT ( .MILLI., .METRE. ) );
#5425=ORIENTED_EDGE ( 'NONE', *, *, #3107, .F. ) ;
#5429=EDGE_CURVE ( 'NONE', #2862, #184, #1177, .T. ) ;
#5433=VECTOR ( 'NONE', #1000, 1000.000000000000000 ) ;
#5437=AXIS2_PLACEMENT_3D ( 'NONE', #6839, #434, #3008 ) ;
#5438=DIRECTION ( 'NONE',  ( 1.000000000000000000, 0.000000000000000000, 0.000000000000000000 ) ) ;
#5453=VERTEX_POINT ( 'NONE', #416 ) ;
#5458=EDGE_CURVE ( 'NONE', #2526, #6097, #2989, .T. ) ;
#5461=VERTEX_POINT ( 'NONE', #2324 ) ;
#5478=ORIENTED_EDGE ( 'NONE', *, *, #1489, .T. ) ;
#5486=LINE ( 'NONE', #4217, #2753 ) ;
#5491=ORIENTED_EDGE ( 'NONE', *, *, #843, .F. ) ;
#5497=DIRECTION ( 'NONE',  ( 0.000000000000000000, 0.000000000000000000, 1.000000000000000000 ) ) ;
#5500=VECTOR ( 'NONE', #4406, 1000.000000000000000 ) ;
#5501=FACE_OUTER_BOUND ( 'NONE', #875, .T. ) ;
#5505=CARTESIAN_POINT ( 'NONE',  ( 80.00000000000000000, 0.000000000000000000, 20.00000000000000000 ) ) ;
#5515=EDGE_CURVE ( 'NONE', #7308, #2526, #6900, .T. ) ;
#5520=CARTESIAN_POINT ( 'NONE',  ( 65.00000000000000000, -12.00000000000000711, 12.49999999999999822 ) ) ;
#5522=EDGE_CURVE ( 'NONE', #731, #7486, #5556, .T. ) ;
#5527=ORIENTED_EDGE ( 'NONE', *, *, #2485, .F. ) ;
#5528=FACE_OUTER_BOUND ( 'NONE', #1062, .T. ) ;
#5538=( NAMED_UNIT ( * ) PLANE_ANGLE_UNIT ( ) SI_UNIT ( $, .RADIAN. ) );
#5548=AXIS2_PLACEMENT_3D ( 'NONE', #7902, #4013, #5358 ) ;
#5556=LINE ( 'NONE', #2568, #5626 ) ;
#5559=AXIS2_PLACEMENT_3D ( 'NONE', #1041, #2391, #4877 ) ;
#5565=ORIENTED_EDGE ( 'NONE', *, *, #5753, .F. ) ;
#5569=CARTESIAN_POINT ( 'NONE',  ( 65.00000000000000000, -7.999999999999996447, 12.49999999999999822 ) ) ;
#5593=LINE ( 'NONE', #5634, #1878 ) ;
#5626=VECTOR ( 'NONE', #6525, 1000.000000000000000 ) ;
#5634=CARTESIAN_POINT ( 'NONE',  ( 80.00000000000000000, 0.000000000000000000, 20.00000000000000000 ) ) ;
#5640=EDGE_CURVE ( 'NONE', #1530, #1162, #578, .T. ) ;
#5656=SURFACE_STYLE_USAGE ( .BOTH. , #399 ) ;
#5658=FACE_BOUND ( 'NONE', #6568, .T. ) ;
#5659=ORIENTED_EDGE ( 'NONE', *, *, #7003, .T. ) ;
#5671=CARTESIAN_POINT ( 'NONE',  ( 47.49999999999999289, -20.00000000000000355, 12.49999999999999112 ) ) ;
#5681=LINE ( 'NONE', #3799, #4030 ) ;
#5682=VERTEX_POINT ( 'NONE', #4449 ) ;
#5692=VECTOR ( 'NONE', #1970, 1000.000000000000000 ) ;
#5697=EDGE_CURVE ( 'NONE', #981, #5461, #3869, .T. ) ;
#5698=DIRECTION ( 'NONE',  ( 1.000000000000000000, -0.000000000000000000, -0.000000000000000000 ) ) ;
#5699=AXIS2_PLACEMENT_3D ( 'NONE', #6884, #2311, #1799 ) ;
#5700=ORIENTED_EDGE ( 'NONE', *, *, #3359, .F. ) ;
#5709=FACE_OUTER_BOUND ( 'NONE', #7229, .T. ) ;
#5712=ADVANCED_FACE ( 'NONE', ( #659, #3242 ), #5798, .T. ) ;
#5715=DIRECTION ( 'NONE',  ( -0.000000000000000000, -0.000000000000000000, -1.000000000000000000 ) ) ;
#5717=ORIENTED_EDGE ( 'NONE', *, *, #6924, .T. ) ;
#5724=EDGE_CURVE ( 'NONE', #731, #4167, #2683, .T. ) ;
#5737=LINE ( 'NONE', #1324, #5031 ) ;
#5749=CARTESIAN_POINT ( 'NONE',  ( -47.50000000000000711, -198.2344135219424857, -12.50000000000005151 ) ) ;
#5753=EDGE_CURVE ( 'NONE', #5461, #7447, #1342, .T. ) ;
#5762=EDGE_CURVE ( 'NONE', #6651, #7734, #747, .T. ) ;
#5769=FACE_OUTER_BOUND ( 'NONE', #6695, .T. ) ;
#5775=DIRECTION ( 'NONE',  ( 0.000000000000000000, -1.734723475976807094E-16, 1.000000000000000000 ) ) ;
#5776=CARTESIAN_POINT ( 'NONE',  ( -47.50000000000002132, -97.00000000000000000, 12.49999999999996803 ) ) ;
#5788=PLANE ( 'NONE',  #8078 ) ;
#5791=CARTESIAN_POINT ( 'NONE',  ( 6.000000000000011546, -100.0010000000000048, -2.499999999999999112 ) ) ;
#5793=DIRECTION ( 'NONE',  ( 1.000000000000000000, 0.000000000000000000, -0.000000000000000000 ) ) ;
#5798=PLANE ( 'NONE',  #4287 ) ;
#5825=CARTESIAN_POINT ( 'NONE',  ( -54.99999999999999289, -97.00000000000000000, 20.00000000000000000 ) ) ;
#5828=AXIS2_PLACEMENT_3D ( 'NONE', #2891, #1627, #948 ) ;
#5830=CARTESIAN_POINT ( 'NONE',  ( -54.99999999999999289, -100.0000000000000000, 20.00000000000000000 ) ) ;
#5832=AXIS2_PLACEMENT_3D ( 'NONE', #1783, #7636, #3127 ) ;
#5845=CARTESIAN_POINT ( 'NONE',  ( 6.000000000000006217, -47.00000000000000000, -2.499999999999999112 ) ) ;
#5856=LINE ( 'NONE', #6536, #2553 ) ;
#5862=CARTESIAN_POINT ( 'NONE',  ( -80.00000000000000000, -20.00000000000000355, 12.49999999999999645 ) ) ;
#5869=FACE_OUTER_BOUND ( 'NONE', #3553, .T. ) ;
#5880=DIRECTION ( 'NONE',  ( 1.000000000000000000, 0.000000000000000000, -0.000000000000000000 ) ) ;
#5896=LINE ( 'NONE', #7717, #1202 ) ;
#5897=EDGE_CURVE ( 'NONE', #2766, #204, #8004, .T. ) ;
#5898=CARTESIAN_POINT ( 'NONE',  ( 65.00000000000000000, -7.999999999999992895, -12.50000000000000178 ) ) ;
#5901=AXIS2_PLACEMENT_3D ( 'NONE', #4533, #7114, #7029 ) ;
#5905=DIRECTION ( 'NONE',  ( 0.000000000000000000, 1.000000000000000000, 0.000000000000000000 ) ) ;
#5915=VECTOR ( 'NONE', #6618, 1000.000000000000000 ) ;
#5943=ADVANCED_FACE ( 'NONE', ( #160 ), #4704, .F. ) ;
#5950=FACE_OUTER_BOUND ( 'NONE', #7464, .T. ) ;
#5954=ORIENTED_EDGE ( 'NONE', *, *, #438, .F. ) ;
#5957=ORIENTED_EDGE ( 'NONE', *, *, #4049, .F. ) ;
#5969=VECTOR ( 'NONE', #764, 1000.000000000000000 ) ;
#5983=AXIS2_PLACEMENT_3D ( 'NONE', #5825, #5154, #5071 ) ;
#5993=LINE ( 'NONE', #976, #3603 ) ;
#5997=ORIENTED_EDGE ( 'NONE', *, *, #7555, .T. ) ;
#6006=LINE ( 'NONE', #2266, #267 ) ;
#6014=ORIENTED_EDGE ( 'NONE', *, *, #2957, .T. ) ;
#6015=DIRECTION ( 'NONE',  ( -0.000000000000000000, -0.7071067811865507924, -0.7071067811865441310 ) ) ;
#6016=PLANE ( 'NONE',  #7321 ) ;
#6034=FACE_OUTER_BOUND ( 'NONE', #2496, .T. ) ;
#6046=CIRCLE ( 'NONE', #7391, 4.000000000000000000 ) ;
#6052=EDGE_LOOP ( 'NONE', ( #3241, #6363, #8136, #5957 ) ) ;
#6075=DIRECTION ( 'NONE',  ( 1.000000000000000000, 1.261617073437677752E-16, 0.000000000000000000 ) ) ;
#6097=VERTEX_POINT ( 'NONE', #4076 ) ;
#6104=CIRCLE ( 'NONE', #5559, 4.000000000000000000 ) ;
#6106=ORIENTED_EDGE ( 'NONE', *, *, #3219, .F. ) ;
#6107=CARTESIAN_POINT ( 'NONE',  ( -47.50000000000000711, -46.99999999999998579, 12.49999999999993960 ) ) ;
#6123=ORIENTED_EDGE ( 'NONE', *, *, #8335, .T. ) ;
#6128=ADVANCED_FACE ( 'NONE', ( #7410, #1551 ), #4115, .F. ) ;
#6131=ORIENTED_EDGE ( 'NONE', *, *, #1253, .T. ) ;
#6132=ADVANCED_FACE ( 'NONE', ( #3451 ), #6727, .T. ) ;
#6134=EDGE_CURVE ( 'NONE', #3662, #7486, #6104, .T. ) ;
#6135=EDGE_LOOP ( 'NONE', ( #2367, #262, #3475, #5116 ) ) ;
#6146=ORIENTED_EDGE ( 'NONE', *, *, #3794, .F. ) ;
#6150=CARTESIAN_POINT ( 'NONE',  ( -5.999999999999988454, -100.0010000000000048, 2.500000000000000888 ) ) ;
#6158=ADVANCED_FACE ( 'NONE', ( #2432 ), #2938, .F. ) ;
#6173=VECTOR ( 'NONE', #1399, 1000.000000000000000 ) ;
#6179=CARTESIAN_POINT ( 'NONE',  ( -47.50000000000002132, -97.00000000000000000, -12.50000000000002309 ) ) ;
#6188=ORIENTED_EDGE ( 'NONE', *, *, #8275, .T. ) ;
#6196=EDGE_CURVE ( 'NONE', #5382, #8240, #8086, .T. ) ;
#6214=ORIENTED_EDGE ( 'NONE', *, *, #2242, .T. ) ;
#6218=EDGE_CURVE ( 'NONE', #1800, #6969, #6932, .T. ) ;
#6220=LINE ( 'NONE', #6179, #2748 ) ;
#6224=VECTOR ( 'NONE', #2543, 1000.000000000000000 ) ;
#6232=PLANE ( 'NONE',  #4413 ) ;
#6243=DIRECTION ( 'NONE',  ( -1.000000000000000000, 0.000000000000000000, -0.000000000000000000 ) ) ;
#6258=EDGE_CURVE ( 'NONE', #1341, #4394, #483, .T. ) ;
#6260=ORIENTED_EDGE ( 'NONE', *, *, #5522, .T. ) ;
#6263=EDGE_CURVE ( 'NONE', #3327, #8040, #6220, .T. ) ;
#6276=LINE ( 'NONE', #2404, #5500 ) ;
#6278=ORIENTED_EDGE ( 'NONE', *, *, #374, .T. ) ;
#6288=ADVANCED_FACE ( 'NONE', ( #3566 ), #361, .T. ) ;
#6296=CARTESIAN_POINT ( 'NONE',  ( 95.11234224026316042, -49.99999999999999289, -20.00000000000000000 ) ) ;
#6297=VECTOR ( 'NONE', #3306, 1000.000000000000000 ) ;
#6301=CARTESIAN_POINT ( 'NONE',  ( -80.00000000000000000, -19.99999999999999645, -12.50000000000000355 ) ) ;
#6303=ORIENTED_EDGE ( 'NONE', *, *, #5184, .F. ) ;
#6345=PLANE ( 'NONE',  #5983 ) ;
#6347=ORIENTED_EDGE ( 'NONE', *, *, #2795, .F. ) ;
#6363=ORIENTED_EDGE ( 'NONE', *, *, #2626, .T. ) ;
#6370=DIRECTION ( 'NONE',  ( 0.000000000000000000, 0.000000000000000000, 1.000000000000000000 ) ) ;
#6385=DIRECTION ( 'NONE',  ( -0.000000000000000000, 1.000000000000000000, 2.775557561562891351E-16 ) ) ;
#6405=ADVANCED_BREP_SHAPE_REPRESENTATION ( '', ( #1832, #2840 ), #4982 ) ;
#6410=LINE ( 'NONE', #170, #6718 ) ;
#6417=LINE ( 'NONE', #1279, #6224 ) ;
#6434=CARTESIAN_POINT ( 'NONE',  ( -80.00000000000000000, -19.99999999999999645, -12.50000000000000000 ) ) ;
#6439=CARTESIAN_POINT ( 'NONE',  ( -5.999999999999992895, -50.00000000000000000, 2.500000000000000888 ) ) ;
#6453=CARTESIAN_POINT ( 'NONE',  ( -3.999999999999988010, -97.00000000000000000, 4.898587196589412829E-16 ) ) ;
#6456=EDGE_CURVE ( 'NONE', #1554, #4845, #2643, .T. ) ;
#6465=VERTEX_POINT ( 'NONE', #688 ) ;
#6467=CARTESIAN_POINT ( 'NONE',  ( 47.49999999999999289, -198.2344135219424857, -12.50000000000005151 ) ) ;
#6471=CARTESIAN_POINT ( 'NONE',  ( -65.00000000000000000, -12.00000000000000711, 12.49999999999999822 ) ) ;
#6474=DIRECTION ( 'NONE',  ( 1.000000000000000000, 9.251858538542971581E-17, -0.000000000000000000 ) ) ;
#6477=CARTESIAN_POINT ( 'NONE',  ( 65.00000000000000000, -12.00000000000000355, -12.50000000000000178 ) ) ;
#6481=DIRECTION ( 'NONE',  ( -1.000000000000000000, -0.000000000000000000, -0.000000000000000000 ) ) ;
#6496=DIRECTION ( 'NONE',  ( 9.251858538542972814E-17, -1.000000000000000000, 0.000000000000000000 ) ) ;
#6500=DIRECTION ( 'NONE',  ( 1.000000000000000000, 2.775557561562892337E-16, -0.000000000000000000 ) ) ;
#6507=PLANE ( 'NONE',  #5156 ) ;
#6508=EDGE_CURVE ( 'NONE', #4681, #2858, #3315, .T. ) ;
#6509=CIRCLE ( 'NONE', #2343, 5.000000000000004441 ) ;
#6510=VECTOR ( 'NONE', #2263, 1000.000000000000000 ) ;
#6523=EDGE_CURVE ( 'NONE', #238, #6651, #3272, .T. ) ;
#6525=DIRECTION ( 'NONE',  ( 1.261617073437677752E-16, -1.000000000000000000, -0.000000000000000000 ) ) ;
#6526=DIRECTION ( 'NONE',  ( 0.000000000000000000, 0.000000000000000000, -1.000000000000000000 ) ) ;
#6536=CARTESIAN_POINT ( 'NONE',  ( 80.00000000000000000, 0.000000000000000000, -20.00000000000000000 ) ) ;
#6542=DIRECTION ( 'NONE',  ( -1.000000000000000000, -1.261617073437677752E-16, 0.000000000000000000 ) ) ;
#6543=DIRECTION ( 'NONE',  ( 1.000000000000000000, 2.775557561562892337E-16, 0.000000000000000000 ) ) ;
#6546=EDGE_LOOP ( 'NONE', ( #3579, #3829, #954, #5327 ) ) ;
#6556=DIRECTION ( 'NONE',  ( 0.000000000000000000, -0.000000000000000000, -1.000000000000000000 ) ) ;
#6558=DIRECTION ( 'NONE',  ( -1.000000000000000000, 8.326672684688674053E-16, 0.000000000000000000 ) ) ;
#6561=EDGE_CURVE ( 'NONE', #1092, #2153, #6509, .T. ) ;
#6563=AXIS2_PLACEMENT_3D ( 'NONE', #2717, #5192, #6542 ) ;
#6566=CARTESIAN_POINT ( 'NONE',  ( -47.50000000000000711, -198.2344135219424857, 12.49999999999993960 ) ) ;
#6568=EDGE_LOOP ( 'NONE', ( #6753, #4126 ) ) ;
#6580=CARTESIAN_POINT ( 'NONE',  ( -80.00000000000000000, 0.000000000000000000, 20.00000000000000000 ) ) ;
#6594=CARTESIAN_POINT ( 'NONE',  ( -80.00000000000000000, -2.168404344971008868E-15, 12.50000000000000000 ) ) ;
#6609=ORIENTED_EDGE ( 'NONE', *, *, #7691, .F. ) ;
#6618=DIRECTION ( 'NONE',  ( -0.000000000000000000, -1.000000000000000000, -0.000000000000000000 ) ) ;
#6623=CARTESIAN_POINT ( 'NONE',  ( 55.00000000000002132, -88.00000000000000000, 0.000000000000000000 ) ) ;
#6626=AXIS2_PLACEMENT_3D ( 'NONE', #7300, #6500, #5233 ) ;
#6638=PLANE ( 'NONE',  #7386 ) ;
#6641=SURFACE_SIDE_STYLE ('',( #1503 ) ) ;
#6651=VERTEX_POINT ( 'NONE', #1245 ) ;
#6658=VERTEX_POINT ( 'NONE', #7694 ) ;
#6664=CARTESIAN_POINT ( 'NONE',  ( -80.00000000000000000, -25.00000000000000000, -20.00000000000000000 ) ) ;
#6668=ORIENTED_EDGE ( 'NONE', *, *, #5697, .F. ) ;
#6674=DIRECTION ( 'NONE',  ( 0.000000000000000000, 0.000000000000000000, 1.000000000000000000 ) ) ;
#6684=DIRECTION ( 'NONE',  ( 2.775557561562892337E-16, -1.000000000000000000, 0.000000000000000000 ) ) ;
#6695=EDGE_LOOP ( 'NONE', ( #3376, #3606, #2283 ) ) ;
#6696=CARTESIAN_POINT ( 'NONE',  ( -80.00000000000000000, 0.000000000000000000, 20.00000000000000000 ) ) ;
#6706=ORIENTED_EDGE ( 'NONE', *, *, #4992, .T. ) ;
#6707=EDGE_CURVE ( 'NONE', #8040, #4798, #14, .T. ) ;
#6718=VECTOR ( 'NONE', #7214, 1000.000000000000000 ) ;
#6719=DIRECTION ( 'NONE',  ( 0.000000000000000000, 0.000000000000000000, -1.000000000000000000 ) ) ;
#6721=FACE_OUTER_BOUND ( 'NONE', #2175, .T. ) ;
#6725=VECTOR ( 'NONE', #3387, 1000.000000000000000 ) ;
#6727=PLANE ( 'NONE',  #1938 ) ;
#6739=DIRECTION ( 'NONE',  ( 1.000000000000000000, 2.775557561562892337E-16, -0.000000000000000000 ) ) ;
#6745=DIRECTION ( 'NONE',  ( -0.000000000000000000, 0.000000000000000000, 1.000000000000000000 ) ) ;
#6753=ORIENTED_EDGE ( 'NONE', *, *, #6134, .F. ) ;
#6775=VECTOR ( 'NONE', #660, 1000.000000000000000 ) ;
#6776=VECTOR ( 'NONE', #4562, 1000.000000000000000 ) ;
#6781=VECTOR ( 'NONE', #4560, 1000.000000000000000 ) ;
#6782=VERTEX_POINT ( 'NONE', #146 ) ;
#6790=PRODUCT_DEFINITION_CONTEXT ( 'detailed design', #2603, 'design' ) ;
#6791=CARTESIAN_POINT ( 'NONE',  ( -55.00000000000000000, -25.00000000000002132, 20.00000000000000000 ) ) ;
#6800=CARTESIAN_POINT ( 'NONE',  ( -65.00000000000000000, -9.999999999999991118, -10.50000000000000888 ) ) ;
#6802=PRESENTATION_STYLE_ASSIGNMENT (( #5656 ) ) ;
#6804=ORIENTED_EDGE ( 'NONE', *, *, #726, .F. ) ;
#6819=PLANE ( 'NONE',  #2014 ) ;
#6820=ORIENTED_EDGE ( 'NONE', *, *, #2281, .F. ) ;
#6828=VECTOR ( 'NONE', #3234, 1000.000000000000000 ) ;
#6829=DIRECTION ( 'NONE',  ( -0.000000000000000000, -0.000000000000000000, -1.000000000000000000 ) ) ;
#6830=ORIENTED_EDGE ( 'NONE', *, *, #5897, .T. ) ;
#6831=DIRECTION ( 'NONE',  ( 0.000000000000000000, -1.000000000000000000, -1.734723475976807094E-16 ) ) ;
#6839=CARTESIAN_POINT ( 'NONE',  ( -5.999999999999988454, -100.0010000000000048, -2.499999999999999112 ) ) ;
#6844=VECTOR ( 'NONE', #91, 1000.000000000000000 ) ;
#6868=DIRECTION ( 'NONE',  ( -2.775557561562892337E-16, 1.000000000000000000, -0.000000000000000000 ) ) ;
#6880=CARTESIAN_POINT ( 'NONE',  ( 65.00000000000000000, -9.999999999999994671, 10.50000000000000533 ) ) ;
#6883=ORIENTED_EDGE ( 'NONE', *, *, #4635, .F. ) ;
#6884=CARTESIAN_POINT ( 'NONE',  ( -47.50000000000000711, -198.2344135219424857, 12.49999999999993960 ) ) ;
#6886=CARTESIAN_POINT ( 'NONE',  ( 1.097606853890779561E-14, -87.00000000000001421, 0.000000000000000000 ) ) ;
#6891=CIRCLE ( 'NONE', #5418, 5.000000000000004441 ) ;
#6900=LINE ( 'NONE', #5671, #5094 ) ;
#6906=AXIS2_PLACEMENT_3D ( 'NONE', #4239, #7448, #1635 ) ;
#6924=EDGE_CURVE ( 'NONE', #5257, #981, #4259, .T. ) ;
#6925=LINE ( 'NONE', #7049, #7985 ) ;
#6931=ORIENTED_EDGE ( 'NONE', *, *, #7520, .F. ) ;
#6932=LINE ( 'NONE', #5505, #3284 ) ;
#6943=EDGE_LOOP ( 'NONE', ( #3708, #7365, #7957, #4889 ) ) ;
#6944=DIRECTION ( 'NONE',  ( -1.000000000000000000, -0.000000000000000000, -0.000000000000000000 ) ) ;
#6946=EDGE_LOOP ( 'NONE', ( #1844, #4815, #234, #493 ) ) ;
#6953=DIRECTION ( 'NONE',  ( -0.000000000000000000, 0.7071067811865484609, 0.7071067811865465735 ) ) ;
#6964=CARTESIAN_POINT ( 'NONE',  ( -80.00000000000000000, 2.168404344971008868E-15, -12.50000000000000000 ) ) ;
#6965=AXIS2_PLACEMENT_3D ( 'NONE', #5318, #1917, #4054 ) ;
#6969=VERTEX_POINT ( 'NONE', #1024 ) ;
#6978=VECTOR ( 'NONE', #6739, 1000.000000000000000 ) ;
#6987=EDGE_LOOP ( 'NONE', ( #3485, #5393, #5058, #5089 ) ) ;
#6998=STYLED_ITEM ( 'NONE', ( #6802 ), #6405 ) ;
#7003=EDGE_CURVE ( 'NONE', #5682, #5004, #982, .T. ) ;
#7010=ADVANCED_FACE ( 'NONE', ( #5528, #3549 ), #4859, .F. ) ;
#7025=FACE_OUTER_BOUND ( 'NONE', #2977, .T. ) ;
#7028=ORIENTED_EDGE ( 'NONE', *, *, #5458, .T. ) ;
#7029=DIRECTION ( 'NONE',  ( -1.000000000000000000, 0.000000000000000000, 0.000000000000000000 ) ) ;
#7048=LINE ( 'NONE', #5862, #6844 ) ;
#7049=CARTESIAN_POINT ( 'NONE',  ( 47.49999999999999289, -46.99999999999998579, 12.49999999999993960 ) ) ;
#7054=VECTOR ( 'NONE', #1412, 1000.000000000000000 ) ;
#7078=EDGE_CURVE ( 'NONE', #2153, #1092, #3428, .T. ) ;
#7083=CARTESIAN_POINT ( 'NONE',  ( 47.49999999999999289, -96.99999999999998579, 12.49999999999996803 ) ) ;
#7087=CARTESIAN_POINT ( 'NONE',  ( -80.00000000000000000, 0.000000000000000000, 20.00000000000000000 ) ) ;
#7090=CARTESIAN_POINT ( 'NONE',  ( 4.000000000000011546, -87.00000000000001421, 0.000000000000000000 ) ) ;
#7091=DIRECTION ( 'NONE',  ( 1.000000000000000000, 9.251858538542971581E-17, 0.000000000000000000 ) ) ;
#7093=SHAPE_REPRESENTATION ( 'High-Rigidity Aluminium Body Shell', ( #2840 ), #4982 ) ;
#7098=ADVANCED_FACE ( 'NONE', ( #1742 ), #3800, .F. ) ;
#7099=FACE_OUTER_BOUND ( 'NONE', #458, .T. ) ;
#7106=DIRECTION ( 'NONE',  ( 0.000000000000000000, -2.775557561562891351E-16, 1.000000000000000000 ) ) ;
#7110=DIRECTION ( 'NONE',  ( -0.000000000000000000, -0.000000000000000000, -1.000000000000000000 ) ) ;
#7113=ORIENTED_EDGE ( 'NONE', *, *, #4472, .F. ) ;
#7114=DIRECTION ( 'NONE',  ( -1.261617073437677752E-16, 1.000000000000000000, 0.000000000000000000 ) ) ;
#7142=ORIENTED_EDGE ( 'NONE', *, *, #3219, .T. ) ;
#7147=DIRECTION ( 'NONE',  ( -1.000000000000000000, -0.000000000000000000, -0.000000000000000000 ) ) ;
#7152=DIRECTION ( 'NONE',  ( 0.000000000000000000, -1.000000000000000000, 0.000000000000000000 ) ) ;
#7162=ORIENTED_EDGE ( 'NONE', *, *, #866, .T. ) ;
#7173=LINE ( 'NONE', #6580, #6173 ) ;
#7184=VERTEX_POINT ( 'NONE', #3000 ) ;
#7186=VECTOR ( 'NONE', #6868, 1000.000000000000000 ) ;
#7187=LINE ( 'NONE', #3313, #49 ) ;
#7192=LINE ( 'NONE', #6471, #1886 ) ;
#7200=VECTOR ( 'NONE', #1633, 1000.000000000000114 ) ;
#7206=ORIENTED_EDGE ( 'NONE', *, *, #438, .T. ) ;
#7214=DIRECTION ( 'NONE',  ( -1.000000000000000000, 0.000000000000000000, 0.000000000000000000 ) ) ;
#7221=DIRECTION ( 'NONE',  ( 1.000000000000000000, 2.775557561562892337E-16, 0.000000000000000000 ) ) ;
#7223=EDGE_CURVE ( 'NONE', #6465, #7540, #1189, .T. ) ;
#7229=EDGE_LOOP ( 'NONE', ( #285, #1285, #7563 ) ) ;
#7244=FACE_BOUND ( 'NONE', #4206, .T. ) ;
#7246=ORIENTED_EDGE ( 'NONE', *, *, #4149, .F. ) ;
#7253=CARTESIAN_POINT ( 'NONE',  ( -47.50000000000000711, -19.99999999999999645, -12.50000000000000355 ) ) ;
#7256=VECTOR ( 'NONE', #3286, 1000.000000000000000 ) ;
#7258=FACE_OUTER_BOUND ( 'NONE', #3285, .T. ) ;
#7259=DIRECTION ( 'NONE',  ( 0.000000000000000000, 1.000000000000000000, 0.000000000000000000 ) ) ;
#7266=ORIENTED_EDGE ( 'NONE', *, *, #508, .F. ) ;
#7281=ORIENTED_EDGE ( 'NONE', *, *, #974, .T. ) ;
#7292=ORIENTED_EDGE ( 'NONE', *, *, #2821, .T. ) ;
#7293=CARTESIAN_POINT ( 'NONE',  ( 65.00000000000000000, -12.00000000000000711, 12.49999999999999822 ) ) ;
#7299=CARTESIAN_POINT ( 'NONE',  ( -54.99999999999999289, -100.0000000000000000, -20.00000000000000000 ) ) ;
#7300=CARTESIAN_POINT ( 'NONE',  ( -80.00100000000001899, -88.00000000000004263, 0.000000000000000000 ) ) ;
#7304=ORIENTED_EDGE ( 'NONE', *, *, #4025, .F. ) ;
#7308=VERTEX_POINT ( 'NONE', #1995 ) ;
#7310=DIRECTION ( 'NONE',  ( 0.000000000000000000, -0.7071067811865484609, 0.7071067811865465735 ) ) ;
#7312=DIRECTION ( 'NONE',  ( 1.000000000000000000, 2.775557561562892337E-16, -0.000000000000000000 ) ) ;
#7318=PRESENTATION_STYLE_ASSIGNMENT (( #2775 ) ) ;
#7321=AXIS2_PLACEMENT_3D ( 'NONE', #792, #4705, #6526 ) ;
#7323=VECTOR ( 'NONE', #6831, 1000.000000000000000 ) ;
#7337=DIRECTION ( 'NONE',  ( -1.261617073437677752E-16, 1.000000000000000000, 0.000000000000000000 ) ) ;
#7351=CARTESIAN_POINT ( 'NONE',  ( 6.000000000000011546, -100.0010000000000048, -2.499999999999999112 ) ) ;
#7365=ORIENTED_EDGE ( 'NONE', *, *, #2654, .F. ) ;
#7371=AXIS2_PLACEMENT_3D ( 'NONE', #5399, #3505, #7980 ) ;
#7374=CARTESIAN_POINT ( 'NONE',  ( -80.00000000000000000, -20.00000000000000355, 12.49999999999999645 ) ) ;
#7378=EDGE_CURVE ( 'NONE', #6969, #1757, #5856, .T. ) ;
#7381=CARTESIAN_POINT ( 'NONE',  ( -5.999999999999993783, -47.00000000000000000, -2.499999999999999112 ) ) ;
#7386=AXIS2_PLACEMENT_3D ( 'NONE', #5791, #6474, #2601 ) ;
#7391=AXIS2_PLACEMENT_3D ( 'NONE', #2750, #7337, #1521 ) ;
#7393=ORIENTED_EDGE ( 'NONE', *, *, #1582, .T. ) ;
#7396=AXIS2_PLACEMENT_3D ( 'NONE', #7597, #1232, #4343 ) ;
#7403=EDGE_CURVE ( 'NONE', #4845, #97, #1355, .T. ) ;
#7406=ORIENTED_EDGE ( 'NONE', *, *, #669, .F. ) ;
#7408=AXIS2_PLACEMENT_3D ( 'NONE', #6150, #4715, #5438 ) ;
#7409=ORIENTED_EDGE ( 'NONE', *, *, #52, .T. ) ;
#7410=FACE_BOUND ( 'NONE', #2680, .T. ) ;
#7413=ORIENTED_EDGE ( 'NONE', *, *, #6263, .F. ) ;
#7421=ORIENTED_EDGE ( 'NONE', *, *, #3472, .F. ) ;
#7422=LINE ( 'NONE', #6107, #3753 ) ;
#7447=VERTEX_POINT ( 'NONE', #2712 ) ;
#7448=DIRECTION ( 'NONE',  ( 0.000000000000000000, -1.734723475976807094E-16, 1.000000000000000000 ) ) ;
#7458=VECTOR ( 'NONE', #2256, 1000.000000000000000 ) ;
#7462=CARTESIAN_POINT ( 'NONE',  ( 47.49999999999999289, -46.99999999999998579, -12.50000000000000888 ) ) ;
#7463=VECTOR ( 'NONE', #6385, 1000.000000000000000 ) ;
#7464=EDGE_LOOP ( 'NONE', ( #1550, #2990, #6123, #8098 ) ) ;
#7474=DIRECTION ( 'NONE',  ( 1.000000000000000000, 9.251858538542971581E-17, 0.000000000000000000 ) ) ;
#7482=FACE_OUTER_BOUND ( 'NONE', #1023, .T. ) ;
#7484=SHAPE_REPRESENTATION_RELATIONSHIP ( 'NONE' , 'NONE' ,  #7093, #6405 ) ;
#7486=VERTEX_POINT ( 'NONE', #6453 ) ;
#7503=ORIENTED_EDGE ( 'NONE', *, *, #2429, .T. ) ;
#7507=DIRECTION ( 'NONE',  ( -1.000000000000000000, -1.261617073437677752E-16, 0.000000000000000000 ) ) ;
#7510=VECTOR ( 'NONE', #4805, 1000.000000000000000 ) ;
#7520=EDGE_CURVE ( 'NONE', #1162, #7447, #807, .T. ) ;
#7523=ORIENTED_EDGE ( 'NONE', *, *, #7520, .T. ) ;
#7540=VERTEX_POINT ( 'NONE', #7253 ) ;
#7541=DIRECTION ( 'NONE',  ( 0.000000000000000000, -0.7071067811865466846, 0.7071067811865484609 ) ) ;
#7550=CARTESIAN_POINT ( 'NONE',  ( -47.50000000000000711, -198.2344135219424857, 12.49999999999993960 ) ) ;
#7555=EDGE_CURVE ( 'NONE', #604, #5453, #1482, .T. ) ;
#7563=ORIENTED_EDGE ( 'NONE', *, *, #7403, .T. ) ;
#7576=ADVANCED_FACE ( 'NONE', ( #5769 ), #3882, .F. ) ;
#7578=CARTESIAN_POINT ( 'NONE',  ( -47.50000000000000711, -97.00000000000000000, 12.49999999999999112 ) ) ;
#7584=VECTOR ( 'NONE', #4100, 1000.000000000000000 ) ;
#7597=CARTESIAN_POINT ( 'NONE',  ( 0.000000000000000000, 0.000000000000000000, -20.00000000000000000 ) ) ;
#7602=DIRECTION ( 'NONE',  ( 0.000000000000000000, -1.000000000000000000, -1.734723475976807094E-16 ) ) ;
#7605=ORIENTED_EDGE ( 'NONE', *, *, #4393, .T. ) ;
#7610=DIRECTION ( 'NONE',  ( 0.000000000000000000, 0.000000000000000000, -1.000000000000000000 ) ) ;
#7623=DIRECTION ( 'NONE',  ( 0.000000000000000000, 2.775557561562892337E-16, -1.000000000000000000 ) ) ;
#7630=ADVANCED_FACE ( 'NONE', ( #1522 ), #2162, .F. ) ;
#7634=EDGE_CURVE ( 'NONE', #6651, #1341, #4890, .T. ) ;
#7636=DIRECTION ( 'NONE',  ( -8.326672684688674053E-16, 1.000000000000000000, 0.000000000000000000 ) ) ;
#7639=CARTESIAN_POINT ( 'NONE',  ( -54.99999999999999289, -100.0000000000000000, 20.00000000000000000 ) ) ;
#7657=CARTESIAN_POINT ( 'NONE',  ( 65.00000000000000000, -7.999999999999992895, -12.50000000000000178 ) ) ;
#7659=VECTOR ( 'NONE', #8175, 1000.000000000000000 ) ;
#7662=DIRECTION ( 'NONE',  ( -0.000000000000000000, 0.000000000000000000, -1.000000000000000000 ) ) ;
#7677=LINE ( 'NONE', #1909, #6978 ) ;
#7691=EDGE_CURVE ( 'NONE', #1798, #5175, #3463, .T. ) ;
#7694=CARTESIAN_POINT ( 'NONE',  ( 47.50000000000000000, -49.99999999999999289, 12.49999999999999289 ) ) ;
#7705=VECTOR ( 'NONE', #7259, 1000.000000000000000 ) ;
#7717=CARTESIAN_POINT ( 'NONE',  ( 80.00000000000000000, -2.168404344971008868E-15, 12.50000000000000000 ) ) ;
#7719=DIRECTION ( 'NONE',  ( 0.000000000000000000, -0.7071067811865484609, 0.7071067811865465735 ) ) ;
#7722=VECTOR ( 'NONE', #5075, 1000.000000000000000 ) ;
#7734=VERTEX_POINT ( 'NONE', #7935 ) ;
#7738=CARTESIAN_POINT ( 'NONE',  ( 47.49999999999999289, -96.99999999999998579, 12.49999999999993960 ) ) ;
#7743=CARTESIAN_POINT ( 'NONE',  ( 80.00000000000000000, -19.99999999999999645, -12.50000000000000355 ) ) ;
#7746=LINE ( 'NONE', #3195, #3058 ) ;
#7751=DIRECTION ( 'NONE',  ( -1.000000000000000000, -9.251858538542971581E-17, 0.000000000000000000 ) ) ;
#7754=ORIENTED_EDGE ( 'NONE', *, *, #3269, .F. ) ;
#7763=CARTESIAN_POINT ( 'NONE',  ( 65.00000000000000000, -7.999999999999992895, -12.50000000000000178 ) ) ;
#7770=PLANE ( 'NONE',  #6563 ) ;
#7777=VECTOR ( 'NONE', #7110, 1000.000000000000000 ) ;
#7779=DIRECTION ( 'NONE',  ( 1.000000000000000000, 8.326672684688674053E-16, -0.000000000000000000 ) ) ;
#7795=CARTESIAN_POINT ( 'NONE',  ( 4.000000000000011546, -87.00000000000001421, 0.000000000000000000 ) ) ;
#7807=PRODUCT_DEFINITION_FORMATION_WITH_SPECIFIED_SOURCE ( 'ANY', '', #4128, .NOT_KNOWN. ) ;
#7814=DIRECTION ( 'NONE',  ( 0.000000000000000000, -1.000000000000000000, -1.734723475976807094E-16 ) ) ;
#7816=VECTOR ( 'NONE', #3211, 1000.000000000000000 ) ;
#7857=FACE_OUTER_BOUND ( 'NONE', #6135, .T. ) ;
#7858=EDGE_CURVE ( 'NONE', #1772, #8255, #7192, .T. ) ;
#7865=ORIENTED_EDGE ( 'NONE', *, *, #6523, .T. ) ;
#7868=LINE ( 'NONE', #2095, #8138 ) ;
#7876=DIRECTION ( 'NONE',  ( -0.000000000000000000, -0.000000000000000000, -1.000000000000000000 ) ) ;
#7883=EDGE_LOOP ( 'NONE', ( #6278, #5659, #6106, #5425, #658, #5171, #4368, #2413 ) ) ;
#7887=ORIENTED_EDGE ( 'NONE', *, *, #1617, .F. ) ;
#7902=CARTESIAN_POINT ( 'NONE',  ( 65.00000000000000000, -12.00000000000000711, 12.49999999999999822 ) ) ;
#7916=DIRECTION ( 'NONE',  ( -1.000000000000000000, -0.000000000000000000, -0.000000000000000000 ) ) ;
#7921=ADVANCED_FACE ( 'NONE', ( #647 ), #5788, .F. ) ;
#7935=CARTESIAN_POINT ( 'NONE',  ( -55.00000000000000000, -25.00000000000002132, 20.00000000000000000 ) ) ;
#7941=CARTESIAN_POINT ( 'NONE',  ( 65.00000000000000000, -12.00000000000000355, -12.50000000000000178 ) ) ;
#7943=VECTOR ( 'NONE', #1577, 1000.000000000000000 ) ;
#7954=DIRECTION ( 'NONE',  ( 0.000000000000000000, -2.775557561562891351E-16, 1.000000000000000000 ) ) ;
#7957=ORIENTED_EDGE ( 'NONE', *, *, #374, .F. ) ;
#7959=CARTESIAN_POINT ( 'NONE',  ( 65.00000000000000000, -7.999999999999996447, 12.49999999999999822 ) ) ;
#7963=ORIENTED_EDGE ( 'NONE', *, *, #2458, .F. ) ;
#7967=ORIENTED_EDGE ( 'NONE', *, *, #5515, .T. ) ;
#7980=DIRECTION ( 'NONE',  ( 0.000000000000000000, 0.000000000000000000, -1.000000000000000000 ) ) ;
#7984=ORIENTED_EDGE ( 'NONE', *, *, #6263, .T. ) ;
#7985=VECTOR ( 'NONE', #2464, 1000.000000000000000 ) ;
#7988=VERTEX_POINT ( 'NONE', #5245 ) ;
#8004=LINE ( 'NONE', #2900, #1331 ) ;
#8007=ORIENTED_EDGE ( 'NONE', *, *, #8144, .F. ) ;
#8016=ORIENTED_EDGE ( 'NONE', *, *, #2821, .F. ) ;
#8017=DIRECTION ( 'NONE',  ( -1.000000000000000000, -9.251858538542971581E-17, 0.000000000000000000 ) ) ;
#8023=LINE ( 'NONE', #2250, #7510 ) ;
#8027=DIRECTION ( 'NONE',  ( -9.251858538542972814E-17, 1.000000000000000000, 0.000000000000000000 ) ) ;
#8029=CARTESIAN_POINT ( 'NONE',  ( -5.999999999999993783, -47.00000000000000000, 2.500000000000000888 ) ) ;
#8036=CARTESIAN_POINT ( 'NONE',  ( 55.00000000000002132, -99.99999999999998579, 20.00000000000000000 ) ) ;
#8040=VERTEX_POINT ( 'NONE', #3985 ) ;
#8043=ORIENTED_EDGE ( 'NONE', *, *, #6924, .F. ) ;
#8044=DIRECTION ( 'NONE',  ( 0.000000000000000000, -1.000000000000000000, 0.000000000000000000 ) ) ;
#8078=AXIS2_PLACEMENT_3D ( 'NONE', #7657, #3317, #5202 ) ;
#8083=COLOUR_RGB ( '', 0.66274510, 0.83137255, 0.94901961) ;
#8086=LINE ( 'NONE', #3651, #5433 ) ;
#8098=ORIENTED_EDGE ( 'NONE', *, *, #3692, .T. ) ;
#8099=CARTESIAN_POINT ( 'NONE',  ( 0.000000000000000000, 0.000000000000000000, 20.00000000000000000 ) ) ;
#8107=ORIENTED_EDGE ( 'NONE', *, *, #6258, .F. ) ;
#8108=CARTESIAN_POINT ( 'NONE',  ( 95.11234224026316042, -46.99999999999999289, -20.00000000000000000 ) ) ;
#8117=LINE ( 'NONE', #312, #2218 ) ;
#8120=CARTESIAN_POINT ( 'NONE',  ( 0.000000000000000000, 0.000000000000000000, 0.000000000000000000 ) ) ;
#8136=ORIENTED_EDGE ( 'NONE', *, *, #3601, .T. ) ;
#8138=VECTOR ( 'NONE', #2136, 1000.000000000000000 ) ;
#8144=EDGE_CURVE ( 'NONE', #97, #1554, #1456, .T. ) ;
#8148=ORIENTED_EDGE ( 'NONE', *, *, #5640, .T. ) ;
#8162=ORIENTED_EDGE ( 'NONE', *, *, #866, .F. ) ;
#8175=DIRECTION ( 'NONE',  ( 1.000000000000000000, -0.000000000000000000, -0.000000000000000000 ) ) ;
#8214=DIRECTION ( 'NONE',  ( 0.000000000000000000, -0.7071067811865483499, -0.7071067811865465735 ) ) ;
#8225=ORIENTED_EDGE ( 'NONE', *, *, #6508, .F. ) ;
#8236=FILL_AREA_STYLE ('',( #3561 ) ) ;
#8240=VERTEX_POINT ( 'NONE', #4733 ) ;
#8254=DIRECTION ( 'NONE',  ( 1.000000000000000000, 9.251858538542971581E-17, 0.000000000000000000 ) ) ;
#8255=VERTEX_POINT ( 'NONE', #4150 ) ;
#8259=VECTOR ( 'NONE', #8254, 1000.000000000000000 ) ;
#8264=VECTOR ( 'NONE', #7602, 1000.000000000000000 ) ;
#8265=LINE ( 'NONE', #1826, #2954 ) ;
#8269=LINE ( 'NONE', #7639, #4689 ) ;
#8272=STYLED_ITEM ( 'NONE', ( #7318 ), #1832 ) ;
#8275=EDGE_CURVE ( 'NONE', #8040, #2655, #6006, .T. ) ;
#8281=EDGE_LOOP ( 'NONE', ( #3539, #4930, #2355, #375 ) ) ;
#8289=VECTOR ( 'NONE', #5189, 1000.000000000000000 ) ;
#8294=CARTESIAN_POINT ( 'NONE',  ( -80.00000000000000000, 2.168404344971008868E-15, -12.50000000000000000 ) ) ;
#8296=ORIENTED_EDGE ( 'NONE', *, *, #4829, .F. ) ;
#8306=ADVANCED_FACE ( 'NONE', ( #6721 ), #952, .T. ) ;
#8314=FACE_OUTER_BOUND ( 'NONE', #1367, .T. ) ;
#8335=EDGE_CURVE ( 'NONE', #1092, #3690, #5414, .T. ) ;
ENDSEC;
END-ISO-10303-21;
